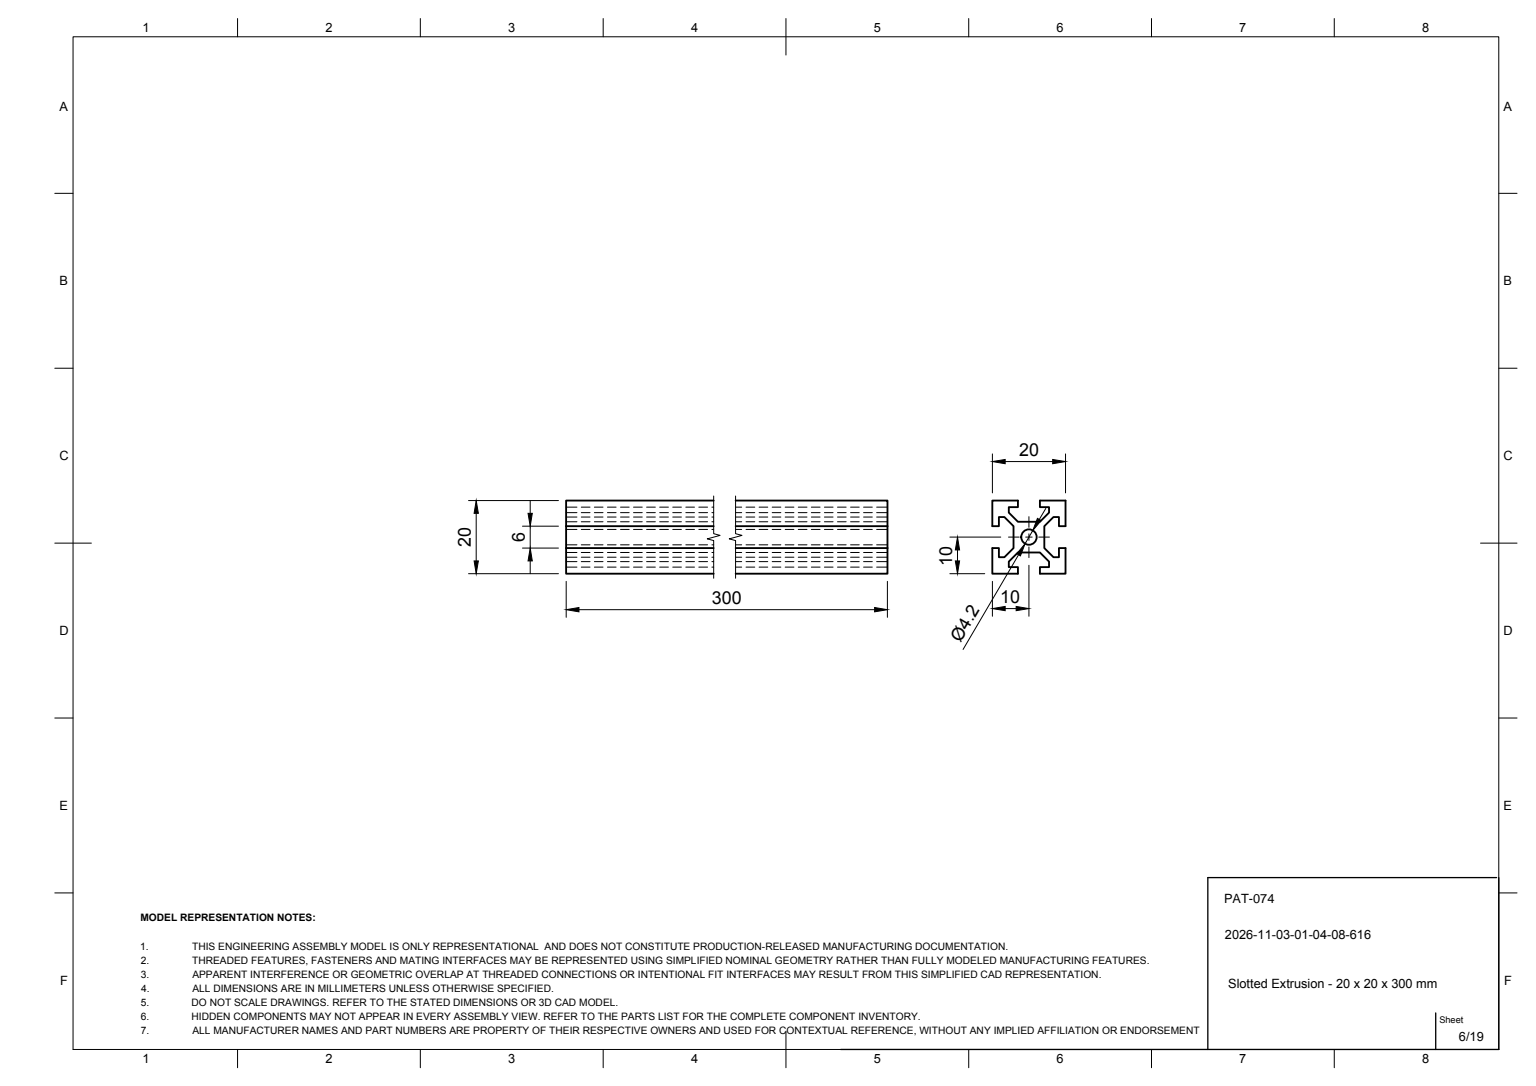
ISO-10303-21;
HEADER;
/* Generated by software containing ST-Developer
 * from STEP Tools, Inc. (www.steptools.com) 
 */

FILE_DESCRIPTION(
/* description */ ('Manual rail carriage with stops'),
/* implementation_level */ '2;1');

FILE_NAME(
/* name */ 'Slotted Extrusion - 20 x 20 x 300 mm.step',
/* time_stamp */ '2026-10-27T18:54:27-07:00',
/* author */ (''),
/* organization */ (''),
/* preprocessor_version */ 'ST-DEVELOPER v20.2',
/* originating_system */ 'Autodesk Translation Framework v15.17.0.0',
/* authorisation */ '');

FILE_SCHEMA (('AUTOMOTIVE_DESIGN { 1 0 10303 214 3 1 1 }'));
ENDSEC;

DATA;
#10=MECHANICAL_DESIGN_GEOMETRIC_PRESENTATION_REPRESENTATION('',(#274),#8499);
#238=SHAPE_REPRESENTATION_RELATIONSHIP('SRR','None',#8601,#256);
#256=ADVANCED_BREP_SHAPE_REPRESENTATION('',(#292),#8480);
#274=STYLED_ITEM('',(#8802),#292);
#292=MANIFOLD_SOLID_BREP('Body1',#4942);
#333=FACE_BOUND('',#936,.T.);
#334=FACE_BOUND('',#938,.T.);
#386=PLANE('',#5214);
#387=PLANE('',#5215);
#388=PLANE('',#5216);
#389=PLANE('',#5217);
#390=PLANE('',#5218);
#391=PLANE('',#5219);
#392=PLANE('',#5220);
#393=PLANE('',#5221);
#394=PLANE('',#5222);
#395=PLANE('',#5223);
#396=PLANE('',#5224);
#397=PLANE('',#5225);
#398=PLANE('',#5226);
#399=PLANE('',#5227);
#400=PLANE('',#5228);
#401=PLANE('',#5229);
#402=PLANE('',#5230);
#403=PLANE('',#5231);
#404=PLANE('',#5232);
#405=PLANE('',#5233);
#406=PLANE('',#5234);
#407=PLANE('',#5235);
#408=PLANE('',#5236);
#409=PLANE('',#5237);
#410=PLANE('',#5238);
#411=PLANE('',#5239);
#412=PLANE('',#5240);
#413=PLANE('',#5241);
#414=PLANE('',#5242);
#415=PLANE('',#5243);
#416=PLANE('',#5244);
#417=PLANE('',#5245);
#418=PLANE('',#5246);
#419=PLANE('',#5247);
#420=PLANE('',#5248);
#421=PLANE('',#5249);
#422=PLANE('',#5253);
#423=PLANE('',#5254);
#424=PLANE('',#5255);
#425=PLANE('',#5256);
#426=PLANE('',#5257);
#427=PLANE('',#5258);
#428=PLANE('',#5259);
#429=PLANE('',#5260);
#430=PLANE('',#5261);
#431=PLANE('',#5262);
#597=FACE_OUTER_BOUND('',#890,.T.);
#598=FACE_OUTER_BOUND('',#891,.T.);
#599=FACE_OUTER_BOUND('',#892,.T.);
#600=FACE_OUTER_BOUND('',#893,.T.);
#601=FACE_OUTER_BOUND('',#894,.T.);
#602=FACE_OUTER_BOUND('',#895,.T.);
#603=FACE_OUTER_BOUND('',#896,.T.);
#604=FACE_OUTER_BOUND('',#897,.T.);
#605=FACE_OUTER_BOUND('',#898,.T.);
#606=FACE_OUTER_BOUND('',#899,.T.);
#607=FACE_OUTER_BOUND('',#900,.T.);
#608=FACE_OUTER_BOUND('',#901,.T.);
#609=FACE_OUTER_BOUND('',#902,.T.);
#610=FACE_OUTER_BOUND('',#903,.T.);
#611=FACE_OUTER_BOUND('',#904,.T.);
#612=FACE_OUTER_BOUND('',#905,.T.);
#613=FACE_OUTER_BOUND('',#906,.T.);
#614=FACE_OUTER_BOUND('',#907,.T.);
#615=FACE_OUTER_BOUND('',#908,.T.);
#616=FACE_OUTER_BOUND('',#909,.T.);
#617=FACE_OUTER_BOUND('',#910,.T.);
#618=FACE_OUTER_BOUND('',#911,.T.);
#619=FACE_OUTER_BOUND('',#912,.T.);
#620=FACE_OUTER_BOUND('',#913,.T.);
#621=FACE_OUTER_BOUND('',#914,.T.);
#622=FACE_OUTER_BOUND('',#915,.T.);
#623=FACE_OUTER_BOUND('',#916,.T.);
#624=FACE_OUTER_BOUND('',#917,.T.);
#625=FACE_OUTER_BOUND('',#918,.T.);
#626=FACE_OUTER_BOUND('',#919,.T.);
#627=FACE_OUTER_BOUND('',#920,.T.);
#628=FACE_OUTER_BOUND('',#921,.T.);
#629=FACE_OUTER_BOUND('',#922,.T.);
#630=FACE_OUTER_BOUND('',#923,.T.);
#631=FACE_OUTER_BOUND('',#924,.T.);
#632=FACE_OUTER_BOUND('',#925,.T.);
#633=FACE_OUTER_BOUND('',#926,.T.);
#634=FACE_OUTER_BOUND('',#927,.T.);
#635=FACE_OUTER_BOUND('',#928,.T.);
#636=FACE_OUTER_BOUND('',#929,.T.);
#637=FACE_OUTER_BOUND('',#930,.T.);
#638=FACE_OUTER_BOUND('',#931,.T.);
#639=FACE_OUTER_BOUND('',#932,.T.);
#640=FACE_OUTER_BOUND('',#933,.T.);
#641=FACE_OUTER_BOUND('',#934,.T.);
#642=FACE_OUTER_BOUND('',#935,.T.);
#643=FACE_OUTER_BOUND('',#937,.T.);
#890=EDGE_LOOP('',(#3468,#3469,#3470,#3471));
#891=EDGE_LOOP('',(#3472,#3473,#3474,#3475));
#892=EDGE_LOOP('',(#3476,#3477,#3478,#3479));
#893=EDGE_LOOP('',(#3480,#3481,#3482,#3483));
#894=EDGE_LOOP('',(#3484,#3485,#3486,#3487));
#895=EDGE_LOOP('',(#3488,#3489,#3490,#3491));
#896=EDGE_LOOP('',(#3492,#3493,#3494,#3495));
#897=EDGE_LOOP('',(#3496,#3497,#3498,#3499));
#898=EDGE_LOOP('',(#3500,#3501,#3502,#3503));
#899=EDGE_LOOP('',(#3504,#3505,#3506,#3507));
#900=EDGE_LOOP('',(#3508,#3509,#3510,#3511));
#901=EDGE_LOOP('',(#3512,#3513,#3514,#3515));
#902=EDGE_LOOP('',(#3516,#3517,#3518,#3519));
#903=EDGE_LOOP('',(#3520,#3521,#3522,#3523));
#904=EDGE_LOOP('',(#3524,#3525,#3526,#3527));
#905=EDGE_LOOP('',(#3528,#3529,#3530,#3531));
#906=EDGE_LOOP('',(#3532,#3533,#3534,#3535));
#907=EDGE_LOOP('',(#3536,#3537,#3538,#3539));
#908=EDGE_LOOP('',(#3540,#3541,#3542,#3543));
#909=EDGE_LOOP('',(#3544,#3545,#3546,#3547));
#910=EDGE_LOOP('',(#3548,#3549,#3550,#3551));
#911=EDGE_LOOP('',(#3552,#3553,#3554,#3555));
#912=EDGE_LOOP('',(#3556,#3557,#3558,#3559));
#913=EDGE_LOOP('',(#3560,#3561,#3562,#3563));
#914=EDGE_LOOP('',(#3564,#3565,#3566,#3567));
#915=EDGE_LOOP('',(#3568,#3569,#3570,#3571));
#916=EDGE_LOOP('',(#3572,#3573,#3574,#3575));
#917=EDGE_LOOP('',(#3576,#3577,#3578,#3579));
#918=EDGE_LOOP('',(#3580,#3581,#3582,#3583));
#919=EDGE_LOOP('',(#3584,#3585,#3586,#3587));
#920=EDGE_LOOP('',(#3588,#3589,#3590,#3591));
#921=EDGE_LOOP('',(#3592,#3593,#3594,#3595));
#922=EDGE_LOOP('',(#3596,#3597,#3598,#3599));
#923=EDGE_LOOP('',(#3600,#3601,#3602,#3603));
#924=EDGE_LOOP('',(#3604,#3605,#3606,#3607));
#925=EDGE_LOOP('',(#3608,#3609,#3610,#3611));
#926=EDGE_LOOP('',(#3612,#3613,#3614,#3615));
#927=EDGE_LOOP('',(#3616,#3617,#3618,#3619));
#928=EDGE_LOOP('',(#3620,#3621,#3622,#3623));
#929=EDGE_LOOP('',(#3624,#3625,#3626,#3627));
#930=EDGE_LOOP('',(#3628,#3629,#3630,#3631));
#931=EDGE_LOOP('',(#3632,#3633,#3634,#3635));
#932=EDGE_LOOP('',(#3636,#3637,#3638,#3639));
#933=EDGE_LOOP('',(#3640,#3641,#3642,#3643));
#934=EDGE_LOOP('',(#3644,#3645,#3646,#3647));
#935=EDGE_LOOP('',(#3648,#3649,#3650,#3651,#3652,#3653,#3654,#3655,#3656,
#3657,#3658,#3659,#3660,#3661,#3662,#3663,#3664,#3665,#3666,#3667,#3668,
#3669,#3670,#3671,#3672,#3673,#3674,#3675,#3676,#3677,#3678,#3679,#3680,
#3681,#3682,#3683,#3684,#3685,#3686,#3687,#3688,#3689,#3690,#3691));
#936=EDGE_LOOP('',(#3692));
#937=EDGE_LOOP('',(#3693,#3694,#3695,#3696,#3697,#3698,#3699,#3700,#3701,
#3702,#3703,#3704,#3705,#3706,#3707,#3708,#3709,#3710,#3711,#3712,#3713,
#3714,#3715,#3716,#3717,#3718,#3719,#3720,#3721,#3722,#3723,#3724,#3725,
#3726,#3727,#3728,#3729,#3730,#3731,#3732,#3733,#3734,#3735,#3736));
#938=EDGE_LOOP('',(#3737));
#1208=LINE('',#7186,#1708);
#1209=LINE('',#7188,#1709);
#1210=LINE('',#7190,#1710);
#1211=LINE('',#7191,#1711);
#1212=LINE('',#7194,#1712);
#1213=LINE('',#7196,#1713);
#1214=LINE('',#7197,#1714);
#1215=LINE('',#7200,#1715);
#1216=LINE('',#7202,#1716);
#1217=LINE('',#7203,#1717);
#1218=LINE('',#7206,#1718);
#1219=LINE('',#7208,#1719);
#1220=LINE('',#7209,#1720);
#1221=LINE('',#7212,#1721);
#1222=LINE('',#7214,#1722);
#1223=LINE('',#7215,#1723);
#1224=LINE('',#7218,#1724);
#1225=LINE('',#7220,#1725);
#1226=LINE('',#7221,#1726);
#1227=LINE('',#7224,#1727);
#1228=LINE('',#7226,#1728);
#1229=LINE('',#7227,#1729);
#1230=LINE('',#7230,#1730);
#1231=LINE('',#7232,#1731);
#1232=LINE('',#7233,#1732);
#1233=LINE('',#7236,#1733);
#1234=LINE('',#7238,#1734);
#1235=LINE('',#7239,#1735);
#1236=LINE('',#7243,#1736);
#1237=LINE('',#7245,#1737);
#1238=LINE('',#7247,#1738);
#1239=LINE('',#7248,#1739);
#1240=LINE('',#7251,#1740);
#1241=LINE('',#7253,#1741);
#1242=LINE('',#7254,#1742);
#1243=LINE('',#7257,#1743);
#1244=LINE('',#7259,#1744);
#1245=LINE('',#7260,#1745);
#1246=LINE('',#7263,#1746);
#1247=LINE('',#7265,#1747);
#1248=LINE('',#7266,#1748);
#1249=LINE('',#7269,#1749);
#1250=LINE('',#7271,#1750);
#1251=LINE('',#7272,#1751);
#1252=LINE('',#7275,#1752);
#1253=LINE('',#7277,#1753);
#1254=LINE('',#7278,#1754);
#1255=LINE('',#7281,#1755);
#1256=LINE('',#7283,#1756);
#1257=LINE('',#7284,#1757);
#1258=LINE('',#7287,#1758);
#1259=LINE('',#7289,#1759);
#1260=LINE('',#7290,#1760);
#1261=LINE('',#7293,#1761);
#1262=LINE('',#7295,#1762);
#1263=LINE('',#7296,#1763);
#1264=LINE('',#7300,#1764);
#1265=LINE('',#7302,#1765);
#1266=LINE('',#7304,#1766);
#1267=LINE('',#7305,#1767);
#1268=LINE('',#7308,#1768);
#1269=LINE('',#7310,#1769);
#1270=LINE('',#7311,#1770);
#1271=LINE('',#7314,#1771);
#1272=LINE('',#7316,#1772);
#1273=LINE('',#7317,#1773);
#1274=LINE('',#7320,#1774);
#1275=LINE('',#7322,#1775);
#1276=LINE('',#7323,#1776);
#1277=LINE('',#7326,#1777);
#1278=LINE('',#7328,#1778);
#1279=LINE('',#7329,#1779);
#1280=LINE('',#7332,#1780);
#1281=LINE('',#7334,#1781);
#1282=LINE('',#7335,#1782);
#1283=LINE('',#7338,#1783);
#1284=LINE('',#7340,#1784);
#1285=LINE('',#7341,#1785);
#1286=LINE('',#7344,#1786);
#1287=LINE('',#7346,#1787);
#1288=LINE('',#7347,#1788);
#1289=LINE('',#7350,#1789);
#1290=LINE('',#7352,#1790);
#1291=LINE('',#7353,#1791);
#1292=LINE('',#7357,#1792);
#1293=LINE('',#7359,#1793);
#1294=LINE('',#7361,#1794);
#1295=LINE('',#7362,#1795);
#1296=LINE('',#7365,#1796);
#1297=LINE('',#7367,#1797);
#1298=LINE('',#7368,#1798);
#1299=LINE('',#7371,#1799);
#1300=LINE('',#7373,#1800);
#1301=LINE('',#7374,#1801);
#1302=LINE('',#7377,#1802);
#1303=LINE('',#7379,#1803);
#1304=LINE('',#7380,#1804);
#1305=LINE('',#7383,#1805);
#1306=LINE('',#7385,#1806);
#1307=LINE('',#7386,#1807);
#1308=LINE('',#7389,#1808);
#1309=LINE('',#7391,#1809);
#1310=LINE('',#7392,#1810);
#1311=LINE('',#7395,#1811);
#1312=LINE('',#7397,#1812);
#1313=LINE('',#7398,#1813);
#1314=LINE('',#7401,#1814);
#1315=LINE('',#7403,#1815);
#1316=LINE('',#7404,#1816);
#1317=LINE('',#7407,#1817);
#1318=LINE('',#7409,#1818);
#1319=LINE('',#7410,#1819);
#1320=LINE('',#7415,#1820);
#1321=LINE('',#7419,#1821);
#1322=LINE('',#7421,#1822);
#1323=LINE('',#7422,#1823);
#1324=LINE('',#7425,#1824);
#1325=LINE('',#7427,#1825);
#1326=LINE('',#7428,#1826);
#1327=LINE('',#7430,#1827);
#1328=LINE('',#7431,#1828);
#1329=LINE('',#7434,#1829);
#1330=LINE('',#7436,#1830);
#1331=LINE('',#7437,#1831);
#1332=LINE('',#7439,#1832);
#1333=LINE('',#7440,#1833);
#1334=LINE('',#7443,#1834);
#1335=LINE('',#7445,#1835);
#1336=LINE('',#7446,#1836);
#1337=LINE('',#7448,#1837);
#1338=LINE('',#7449,#1838);
#1339=LINE('',#7451,#1839);
#1340=LINE('',#7452,#1840);
#1708=VECTOR('',#5763,1.);
#1709=VECTOR('',#5764,1.);
#1710=VECTOR('',#5765,1.);
#1711=VECTOR('',#5766,1.);
#1712=VECTOR('',#5769,1.);
#1713=VECTOR('',#5770,1.);
#1714=VECTOR('',#5771,1.);
#1715=VECTOR('',#5774,1.);
#1716=VECTOR('',#5775,1.);
#1717=VECTOR('',#5776,1.);
#1718=VECTOR('',#5779,1.);
#1719=VECTOR('',#5780,1.);
#1720=VECTOR('',#5781,1.);
#1721=VECTOR('',#5784,1.);
#1722=VECTOR('',#5785,1.);
#1723=VECTOR('',#5786,1.);
#1724=VECTOR('',#5789,1.);
#1725=VECTOR('',#5790,1.);
#1726=VECTOR('',#5791,1.);
#1727=VECTOR('',#5794,1.);
#1728=VECTOR('',#5795,1.);
#1729=VECTOR('',#5796,1.);
#1730=VECTOR('',#5799,1.);
#1731=VECTOR('',#5800,1.);
#1732=VECTOR('',#5801,1.);
#1733=VECTOR('',#5804,1.);
#1734=VECTOR('',#5805,1.);
#1735=VECTOR('',#5806,1.);
#1736=VECTOR('',#5809,1.);
#1737=VECTOR('',#5810,1.);
#1738=VECTOR('',#5811,1.);
#1739=VECTOR('',#5812,1.);
#1740=VECTOR('',#5815,1.);
#1741=VECTOR('',#5816,1.);
#1742=VECTOR('',#5817,1.);
#1743=VECTOR('',#5820,1.);
#1744=VECTOR('',#5821,1.);
#1745=VECTOR('',#5822,1.);
#1746=VECTOR('',#5825,1.);
#1747=VECTOR('',#5826,1.);
#1748=VECTOR('',#5827,1.);
#1749=VECTOR('',#5830,1.);
#1750=VECTOR('',#5831,1.);
#1751=VECTOR('',#5832,1.);
#1752=VECTOR('',#5835,1.);
#1753=VECTOR('',#5836,1.);
#1754=VECTOR('',#5837,1.);
#1755=VECTOR('',#5840,1.);
#1756=VECTOR('',#5841,1.);
#1757=VECTOR('',#5842,1.);
#1758=VECTOR('',#5845,1.);
#1759=VECTOR('',#5846,1.);
#1760=VECTOR('',#5847,1.);
#1761=VECTOR('',#5850,1.);
#1762=VECTOR('',#5851,1.);
#1763=VECTOR('',#5852,1.);
#1764=VECTOR('',#5855,1.);
#1765=VECTOR('',#5856,1.);
#1766=VECTOR('',#5857,1.);
#1767=VECTOR('',#5858,1.);
#1768=VECTOR('',#5861,1.);
#1769=VECTOR('',#5862,1.);
#1770=VECTOR('',#5863,1.);
#1771=VECTOR('',#5866,1.);
#1772=VECTOR('',#5867,1.);
#1773=VECTOR('',#5868,1.);
#1774=VECTOR('',#5871,1.);
#1775=VECTOR('',#5872,1.);
#1776=VECTOR('',#5873,1.);
#1777=VECTOR('',#5876,1.);
#1778=VECTOR('',#5877,1.);
#1779=VECTOR('',#5878,1.);
#1780=VECTOR('',#5881,1.);
#1781=VECTOR('',#5882,1.);
#1782=VECTOR('',#5883,1.);
#1783=VECTOR('',#5886,1.);
#1784=VECTOR('',#5887,1.);
#1785=VECTOR('',#5888,1.);
#1786=VECTOR('',#5891,1.);
#1787=VECTOR('',#5892,1.);
#1788=VECTOR('',#5893,1.);
#1789=VECTOR('',#5896,1.);
#1790=VECTOR('',#5897,1.);
#1791=VECTOR('',#5898,1.);
#1792=VECTOR('',#5901,1.);
#1793=VECTOR('',#5902,1.);
#1794=VECTOR('',#5903,1.);
#1795=VECTOR('',#5904,1.);
#1796=VECTOR('',#5907,1.);
#1797=VECTOR('',#5908,1.);
#1798=VECTOR('',#5909,1.);
#1799=VECTOR('',#5912,1.);
#1800=VECTOR('',#5913,1.);
#1801=VECTOR('',#5914,1.);
#1802=VECTOR('',#5917,1.);
#1803=VECTOR('',#5918,1.);
#1804=VECTOR('',#5919,1.);
#1805=VECTOR('',#5922,1.);
#1806=VECTOR('',#5923,1.);
#1807=VECTOR('',#5924,1.);
#1808=VECTOR('',#5927,1.);
#1809=VECTOR('',#5928,1.);
#1810=VECTOR('',#5929,1.);
#1811=VECTOR('',#5932,1.);
#1812=VECTOR('',#5933,1.);
#1813=VECTOR('',#5934,1.);
#1814=VECTOR('',#5937,1.);
#1815=VECTOR('',#5938,1.);
#1816=VECTOR('',#5939,1.);
#1817=VECTOR('',#5942,1.);
#1818=VECTOR('',#5943,1.);
#1819=VECTOR('',#5944,1.);
#1820=VECTOR('',#5949,0.21);
#1821=VECTOR('',#5954,1.);
#1822=VECTOR('',#5955,1.);
#1823=VECTOR('',#5956,1.);
#1824=VECTOR('',#5959,1.);
#1825=VECTOR('',#5960,1.);
#1826=VECTOR('',#5961,1.);
#1827=VECTOR('',#5964,1.);
#1828=VECTOR('',#5965,1.);
#1829=VECTOR('',#5968,1.);
#1830=VECTOR('',#5969,1.);
#1831=VECTOR('',#5970,1.);
#1832=VECTOR('',#5973,1.);
#1833=VECTOR('',#5974,1.);
#1834=VECTOR('',#5977,1.);
#1835=VECTOR('',#5978,1.);
#1836=VECTOR('',#5979,1.);
#1837=VECTOR('',#5982,1.);
#1838=VECTOR('',#5983,1.);
#1839=VECTOR('',#5986,1.);
#1840=VECTOR('',#5987,1.);
#2210=CIRCLE('',#5251,0.21);
#2211=CIRCLE('',#5252,0.21);
#2348=VERTEX_POINT('',#7184);
#2349=VERTEX_POINT('',#7185);
#2350=VERTEX_POINT('',#7187);
#2351=VERTEX_POINT('',#7189);
#2352=VERTEX_POINT('',#7193);
#2353=VERTEX_POINT('',#7195);
#2354=VERTEX_POINT('',#7199);
#2355=VERTEX_POINT('',#7201);
#2356=VERTEX_POINT('',#7205);
#2357=VERTEX_POINT('',#7207);
#2358=VERTEX_POINT('',#7211);
#2359=VERTEX_POINT('',#7213);
#2360=VERTEX_POINT('',#7217);
#2361=VERTEX_POINT('',#7219);
#2362=VERTEX_POINT('',#7223);
#2363=VERTEX_POINT('',#7225);
#2364=VERTEX_POINT('',#7229);
#2365=VERTEX_POINT('',#7231);
#2366=VERTEX_POINT('',#7235);
#2367=VERTEX_POINT('',#7237);
#2368=VERTEX_POINT('',#7241);
#2369=VERTEX_POINT('',#7242);
#2370=VERTEX_POINT('',#7244);
#2371=VERTEX_POINT('',#7246);
#2372=VERTEX_POINT('',#7250);
#2373=VERTEX_POINT('',#7252);
#2374=VERTEX_POINT('',#7256);
#2375=VERTEX_POINT('',#7258);
#2376=VERTEX_POINT('',#7262);
#2377=VERTEX_POINT('',#7264);
#2378=VERTEX_POINT('',#7268);
#2379=VERTEX_POINT('',#7270);
#2380=VERTEX_POINT('',#7274);
#2381=VERTEX_POINT('',#7276);
#2382=VERTEX_POINT('',#7280);
#2383=VERTEX_POINT('',#7282);
#2384=VERTEX_POINT('',#7286);
#2385=VERTEX_POINT('',#7288);
#2386=VERTEX_POINT('',#7292);
#2387=VERTEX_POINT('',#7294);
#2388=VERTEX_POINT('',#7298);
#2389=VERTEX_POINT('',#7299);
#2390=VERTEX_POINT('',#7301);
#2391=VERTEX_POINT('',#7303);
#2392=VERTEX_POINT('',#7307);
#2393=VERTEX_POINT('',#7309);
#2394=VERTEX_POINT('',#7313);
#2395=VERTEX_POINT('',#7315);
#2396=VERTEX_POINT('',#7319);
#2397=VERTEX_POINT('',#7321);
#2398=VERTEX_POINT('',#7325);
#2399=VERTEX_POINT('',#7327);
#2400=VERTEX_POINT('',#7331);
#2401=VERTEX_POINT('',#7333);
#2402=VERTEX_POINT('',#7337);
#2403=VERTEX_POINT('',#7339);
#2404=VERTEX_POINT('',#7343);
#2405=VERTEX_POINT('',#7345);
#2406=VERTEX_POINT('',#7349);
#2407=VERTEX_POINT('',#7351);
#2408=VERTEX_POINT('',#7355);
#2409=VERTEX_POINT('',#7356);
#2410=VERTEX_POINT('',#7358);
#2411=VERTEX_POINT('',#7360);
#2412=VERTEX_POINT('',#7364);
#2413=VERTEX_POINT('',#7366);
#2414=VERTEX_POINT('',#7370);
#2415=VERTEX_POINT('',#7372);
#2416=VERTEX_POINT('',#7376);
#2417=VERTEX_POINT('',#7378);
#2418=VERTEX_POINT('',#7382);
#2419=VERTEX_POINT('',#7384);
#2420=VERTEX_POINT('',#7388);
#2421=VERTEX_POINT('',#7390);
#2422=VERTEX_POINT('',#7394);
#2423=VERTEX_POINT('',#7396);
#2424=VERTEX_POINT('',#7400);
#2425=VERTEX_POINT('',#7402);
#2426=VERTEX_POINT('',#7406);
#2427=VERTEX_POINT('',#7408);
#2428=VERTEX_POINT('',#7412);
#2429=VERTEX_POINT('',#7414);
#2430=VERTEX_POINT('',#7418);
#2431=VERTEX_POINT('',#7420);
#2432=VERTEX_POINT('',#7424);
#2433=VERTEX_POINT('',#7426);
#2434=VERTEX_POINT('',#7433);
#2435=VERTEX_POINT('',#7435);
#2436=VERTEX_POINT('',#7442);
#2437=VERTEX_POINT('',#7444);
#2782=EDGE_CURVE('',#2348,#2349,#1208,.T.);
#2783=EDGE_CURVE('',#2348,#2350,#1209,.T.);
#2784=EDGE_CURVE('',#2351,#2350,#1210,.T.);
#2785=EDGE_CURVE('',#2349,#2351,#1211,.T.);
#2786=EDGE_CURVE('',#2352,#2348,#1212,.T.);
#2787=EDGE_CURVE('',#2352,#2353,#1213,.T.);
#2788=EDGE_CURVE('',#2350,#2353,#1214,.T.);
#2789=EDGE_CURVE('',#2354,#2352,#1215,.T.);
#2790=EDGE_CURVE('',#2354,#2355,#1216,.T.);
#2791=EDGE_CURVE('',#2353,#2355,#1217,.T.);
#2792=EDGE_CURVE('',#2356,#2354,#1218,.T.);
#2793=EDGE_CURVE('',#2356,#2357,#1219,.T.);
#2794=EDGE_CURVE('',#2355,#2357,#1220,.T.);
#2795=EDGE_CURVE('',#2358,#2356,#1221,.T.);
#2796=EDGE_CURVE('',#2358,#2359,#1222,.T.);
#2797=EDGE_CURVE('',#2357,#2359,#1223,.T.);
#2798=EDGE_CURVE('',#2360,#2358,#1224,.T.);
#2799=EDGE_CURVE('',#2360,#2361,#1225,.T.);
#2800=EDGE_CURVE('',#2359,#2361,#1226,.T.);
#2801=EDGE_CURVE('',#2362,#2360,#1227,.T.);
#2802=EDGE_CURVE('',#2362,#2363,#1228,.T.);
#2803=EDGE_CURVE('',#2361,#2363,#1229,.T.);
#2804=EDGE_CURVE('',#2364,#2362,#1230,.T.);
#2805=EDGE_CURVE('',#2364,#2365,#1231,.T.);
#2806=EDGE_CURVE('',#2363,#2365,#1232,.T.);
#2807=EDGE_CURVE('',#2366,#2364,#1233,.T.);
#2808=EDGE_CURVE('',#2367,#2366,#1234,.T.);
#2809=EDGE_CURVE('',#2365,#2367,#1235,.T.);
#2810=EDGE_CURVE('',#2368,#2369,#1236,.T.);
#2811=EDGE_CURVE('',#2368,#2370,#1237,.T.);
#2812=EDGE_CURVE('',#2371,#2370,#1238,.T.);
#2813=EDGE_CURVE('',#2369,#2371,#1239,.T.);
#2814=EDGE_CURVE('',#2372,#2368,#1240,.T.);
#2815=EDGE_CURVE('',#2372,#2373,#1241,.T.);
#2816=EDGE_CURVE('',#2370,#2373,#1242,.T.);
#2817=EDGE_CURVE('',#2374,#2372,#1243,.T.);
#2818=EDGE_CURVE('',#2374,#2375,#1244,.T.);
#2819=EDGE_CURVE('',#2373,#2375,#1245,.T.);
#2820=EDGE_CURVE('',#2376,#2374,#1246,.T.);
#2821=EDGE_CURVE('',#2376,#2377,#1247,.T.);
#2822=EDGE_CURVE('',#2375,#2377,#1248,.T.);
#2823=EDGE_CURVE('',#2378,#2376,#1249,.T.);
#2824=EDGE_CURVE('',#2378,#2379,#1250,.T.);
#2825=EDGE_CURVE('',#2377,#2379,#1251,.T.);
#2826=EDGE_CURVE('',#2380,#2378,#1252,.T.);
#2827=EDGE_CURVE('',#2380,#2381,#1253,.T.);
#2828=EDGE_CURVE('',#2379,#2381,#1254,.T.);
#2829=EDGE_CURVE('',#2382,#2380,#1255,.T.);
#2830=EDGE_CURVE('',#2382,#2383,#1256,.T.);
#2831=EDGE_CURVE('',#2381,#2383,#1257,.T.);
#2832=EDGE_CURVE('',#2384,#2382,#1258,.T.);
#2833=EDGE_CURVE('',#2384,#2385,#1259,.T.);
#2834=EDGE_CURVE('',#2383,#2385,#1260,.T.);
#2835=EDGE_CURVE('',#2386,#2384,#1261,.T.);
#2836=EDGE_CURVE('',#2387,#2386,#1262,.T.);
#2837=EDGE_CURVE('',#2385,#2387,#1263,.T.);
#2838=EDGE_CURVE('',#2388,#2389,#1264,.T.);
#2839=EDGE_CURVE('',#2388,#2390,#1265,.T.);
#2840=EDGE_CURVE('',#2391,#2390,#1266,.T.);
#2841=EDGE_CURVE('',#2389,#2391,#1267,.T.);
#2842=EDGE_CURVE('',#2392,#2388,#1268,.T.);
#2843=EDGE_CURVE('',#2392,#2393,#1269,.T.);
#2844=EDGE_CURVE('',#2390,#2393,#1270,.T.);
#2845=EDGE_CURVE('',#2394,#2392,#1271,.T.);
#2846=EDGE_CURVE('',#2394,#2395,#1272,.T.);
#2847=EDGE_CURVE('',#2393,#2395,#1273,.T.);
#2848=EDGE_CURVE('',#2396,#2394,#1274,.T.);
#2849=EDGE_CURVE('',#2396,#2397,#1275,.T.);
#2850=EDGE_CURVE('',#2395,#2397,#1276,.T.);
#2851=EDGE_CURVE('',#2398,#2396,#1277,.T.);
#2852=EDGE_CURVE('',#2398,#2399,#1278,.T.);
#2853=EDGE_CURVE('',#2397,#2399,#1279,.T.);
#2854=EDGE_CURVE('',#2400,#2398,#1280,.T.);
#2855=EDGE_CURVE('',#2400,#2401,#1281,.T.);
#2856=EDGE_CURVE('',#2399,#2401,#1282,.T.);
#2857=EDGE_CURVE('',#2402,#2400,#1283,.T.);
#2858=EDGE_CURVE('',#2402,#2403,#1284,.T.);
#2859=EDGE_CURVE('',#2401,#2403,#1285,.T.);
#2860=EDGE_CURVE('',#2404,#2402,#1286,.T.);
#2861=EDGE_CURVE('',#2404,#2405,#1287,.T.);
#2862=EDGE_CURVE('',#2403,#2405,#1288,.T.);
#2863=EDGE_CURVE('',#2406,#2404,#1289,.T.);
#2864=EDGE_CURVE('',#2407,#2406,#1290,.T.);
#2865=EDGE_CURVE('',#2405,#2407,#1291,.T.);
#2866=EDGE_CURVE('',#2408,#2409,#1292,.T.);
#2867=EDGE_CURVE('',#2408,#2410,#1293,.T.);
#2868=EDGE_CURVE('',#2411,#2410,#1294,.T.);
#2869=EDGE_CURVE('',#2409,#2411,#1295,.T.);
#2870=EDGE_CURVE('',#2412,#2408,#1296,.T.);
#2871=EDGE_CURVE('',#2412,#2413,#1297,.T.);
#2872=EDGE_CURVE('',#2410,#2413,#1298,.T.);
#2873=EDGE_CURVE('',#2414,#2412,#1299,.T.);
#2874=EDGE_CURVE('',#2414,#2415,#1300,.T.);
#2875=EDGE_CURVE('',#2413,#2415,#1301,.T.);
#2876=EDGE_CURVE('',#2416,#2414,#1302,.T.);
#2877=EDGE_CURVE('',#2416,#2417,#1303,.T.);
#2878=EDGE_CURVE('',#2415,#2417,#1304,.T.);
#2879=EDGE_CURVE('',#2418,#2416,#1305,.T.);
#2880=EDGE_CURVE('',#2418,#2419,#1306,.T.);
#2881=EDGE_CURVE('',#2417,#2419,#1307,.T.);
#2882=EDGE_CURVE('',#2420,#2418,#1308,.T.);
#2883=EDGE_CURVE('',#2420,#2421,#1309,.T.);
#2884=EDGE_CURVE('',#2419,#2421,#1310,.T.);
#2885=EDGE_CURVE('',#2422,#2420,#1311,.T.);
#2886=EDGE_CURVE('',#2422,#2423,#1312,.T.);
#2887=EDGE_CURVE('',#2421,#2423,#1313,.T.);
#2888=EDGE_CURVE('',#2424,#2422,#1314,.T.);
#2889=EDGE_CURVE('',#2424,#2425,#1315,.T.);
#2890=EDGE_CURVE('',#2423,#2425,#1316,.T.);
#2891=EDGE_CURVE('',#2426,#2424,#1317,.T.);
#2892=EDGE_CURVE('',#2427,#2426,#1318,.T.);
#2893=EDGE_CURVE('',#2425,#2427,#1319,.T.);
#2894=EDGE_CURVE('',#2428,#2428,#2210,.T.);
#2895=EDGE_CURVE('',#2428,#2429,#1320,.T.);
#2896=EDGE_CURVE('',#2429,#2429,#2211,.T.);
#2897=EDGE_CURVE('',#2366,#2430,#1321,.T.);
#2898=EDGE_CURVE('',#2430,#2431,#1322,.T.);
#2899=EDGE_CURVE('',#2367,#2431,#1323,.T.);
#2900=EDGE_CURVE('',#2432,#2351,#1324,.T.);
#2901=EDGE_CURVE('',#2433,#2432,#1325,.T.);
#2902=EDGE_CURVE('',#2433,#2349,#1326,.T.);
#2903=EDGE_CURVE('',#2386,#2433,#1327,.T.);
#2904=EDGE_CURVE('',#2387,#2432,#1328,.T.);
#2905=EDGE_CURVE('',#2434,#2371,#1329,.T.);
#2906=EDGE_CURVE('',#2435,#2434,#1330,.T.);
#2907=EDGE_CURVE('',#2435,#2369,#1331,.T.);
#2908=EDGE_CURVE('',#2406,#2435,#1332,.T.);
#2909=EDGE_CURVE('',#2407,#2434,#1333,.T.);
#2910=EDGE_CURVE('',#2436,#2391,#1334,.T.);
#2911=EDGE_CURVE('',#2437,#2436,#1335,.T.);
#2912=EDGE_CURVE('',#2437,#2389,#1336,.T.);
#2913=EDGE_CURVE('',#2426,#2437,#1337,.T.);
#2914=EDGE_CURVE('',#2427,#2436,#1338,.T.);
#2915=EDGE_CURVE('',#2431,#2411,#1339,.T.);
#2916=EDGE_CURVE('',#2430,#2409,#1340,.T.);
#3468=ORIENTED_EDGE('',*,*,#2782,.F.);
#3469=ORIENTED_EDGE('',*,*,#2783,.T.);
#3470=ORIENTED_EDGE('',*,*,#2784,.F.);
#3471=ORIENTED_EDGE('',*,*,#2785,.F.);
#3472=ORIENTED_EDGE('',*,*,#2786,.F.);
#3473=ORIENTED_EDGE('',*,*,#2787,.T.);
#3474=ORIENTED_EDGE('',*,*,#2788,.F.);
#3475=ORIENTED_EDGE('',*,*,#2783,.F.);
#3476=ORIENTED_EDGE('',*,*,#2789,.F.);
#3477=ORIENTED_EDGE('',*,*,#2790,.T.);
#3478=ORIENTED_EDGE('',*,*,#2791,.F.);
#3479=ORIENTED_EDGE('',*,*,#2787,.F.);
#3480=ORIENTED_EDGE('',*,*,#2792,.F.);
#3481=ORIENTED_EDGE('',*,*,#2793,.T.);
#3482=ORIENTED_EDGE('',*,*,#2794,.F.);
#3483=ORIENTED_EDGE('',*,*,#2790,.F.);
#3484=ORIENTED_EDGE('',*,*,#2795,.F.);
#3485=ORIENTED_EDGE('',*,*,#2796,.T.);
#3486=ORIENTED_EDGE('',*,*,#2797,.F.);
#3487=ORIENTED_EDGE('',*,*,#2793,.F.);
#3488=ORIENTED_EDGE('',*,*,#2798,.F.);
#3489=ORIENTED_EDGE('',*,*,#2799,.T.);
#3490=ORIENTED_EDGE('',*,*,#2800,.F.);
#3491=ORIENTED_EDGE('',*,*,#2796,.F.);
#3492=ORIENTED_EDGE('',*,*,#2801,.F.);
#3493=ORIENTED_EDGE('',*,*,#2802,.T.);
#3494=ORIENTED_EDGE('',*,*,#2803,.F.);
#3495=ORIENTED_EDGE('',*,*,#2799,.F.);
#3496=ORIENTED_EDGE('',*,*,#2804,.F.);
#3497=ORIENTED_EDGE('',*,*,#2805,.T.);
#3498=ORIENTED_EDGE('',*,*,#2806,.F.);
#3499=ORIENTED_EDGE('',*,*,#2802,.F.);
#3500=ORIENTED_EDGE('',*,*,#2807,.F.);
#3501=ORIENTED_EDGE('',*,*,#2808,.F.);
#3502=ORIENTED_EDGE('',*,*,#2809,.F.);
#3503=ORIENTED_EDGE('',*,*,#2805,.F.);
#3504=ORIENTED_EDGE('',*,*,#2810,.F.);
#3505=ORIENTED_EDGE('',*,*,#2811,.T.);
#3506=ORIENTED_EDGE('',*,*,#2812,.F.);
#3507=ORIENTED_EDGE('',*,*,#2813,.F.);
#3508=ORIENTED_EDGE('',*,*,#2814,.F.);
#3509=ORIENTED_EDGE('',*,*,#2815,.T.);
#3510=ORIENTED_EDGE('',*,*,#2816,.F.);
#3511=ORIENTED_EDGE('',*,*,#2811,.F.);
#3512=ORIENTED_EDGE('',*,*,#2817,.F.);
#3513=ORIENTED_EDGE('',*,*,#2818,.T.);
#3514=ORIENTED_EDGE('',*,*,#2819,.F.);
#3515=ORIENTED_EDGE('',*,*,#2815,.F.);
#3516=ORIENTED_EDGE('',*,*,#2820,.F.);
#3517=ORIENTED_EDGE('',*,*,#2821,.T.);
#3518=ORIENTED_EDGE('',*,*,#2822,.F.);
#3519=ORIENTED_EDGE('',*,*,#2818,.F.);
#3520=ORIENTED_EDGE('',*,*,#2823,.F.);
#3521=ORIENTED_EDGE('',*,*,#2824,.T.);
#3522=ORIENTED_EDGE('',*,*,#2825,.F.);
#3523=ORIENTED_EDGE('',*,*,#2821,.F.);
#3524=ORIENTED_EDGE('',*,*,#2826,.F.);
#3525=ORIENTED_EDGE('',*,*,#2827,.T.);
#3526=ORIENTED_EDGE('',*,*,#2828,.F.);
#3527=ORIENTED_EDGE('',*,*,#2824,.F.);
#3528=ORIENTED_EDGE('',*,*,#2829,.F.);
#3529=ORIENTED_EDGE('',*,*,#2830,.T.);
#3530=ORIENTED_EDGE('',*,*,#2831,.F.);
#3531=ORIENTED_EDGE('',*,*,#2827,.F.);
#3532=ORIENTED_EDGE('',*,*,#2832,.F.);
#3533=ORIENTED_EDGE('',*,*,#2833,.T.);
#3534=ORIENTED_EDGE('',*,*,#2834,.F.);
#3535=ORIENTED_EDGE('',*,*,#2830,.F.);
#3536=ORIENTED_EDGE('',*,*,#2835,.F.);
#3537=ORIENTED_EDGE('',*,*,#2836,.F.);
#3538=ORIENTED_EDGE('',*,*,#2837,.F.);
#3539=ORIENTED_EDGE('',*,*,#2833,.F.);
#3540=ORIENTED_EDGE('',*,*,#2838,.F.);
#3541=ORIENTED_EDGE('',*,*,#2839,.T.);
#3542=ORIENTED_EDGE('',*,*,#2840,.F.);
#3543=ORIENTED_EDGE('',*,*,#2841,.F.);
#3544=ORIENTED_EDGE('',*,*,#2842,.F.);
#3545=ORIENTED_EDGE('',*,*,#2843,.T.);
#3546=ORIENTED_EDGE('',*,*,#2844,.F.);
#3547=ORIENTED_EDGE('',*,*,#2839,.F.);
#3548=ORIENTED_EDGE('',*,*,#2845,.F.);
#3549=ORIENTED_EDGE('',*,*,#2846,.T.);
#3550=ORIENTED_EDGE('',*,*,#2847,.F.);
#3551=ORIENTED_EDGE('',*,*,#2843,.F.);
#3552=ORIENTED_EDGE('',*,*,#2848,.F.);
#3553=ORIENTED_EDGE('',*,*,#2849,.T.);
#3554=ORIENTED_EDGE('',*,*,#2850,.F.);
#3555=ORIENTED_EDGE('',*,*,#2846,.F.);
#3556=ORIENTED_EDGE('',*,*,#2851,.F.);
#3557=ORIENTED_EDGE('',*,*,#2852,.T.);
#3558=ORIENTED_EDGE('',*,*,#2853,.F.);
#3559=ORIENTED_EDGE('',*,*,#2849,.F.);
#3560=ORIENTED_EDGE('',*,*,#2854,.F.);
#3561=ORIENTED_EDGE('',*,*,#2855,.T.);
#3562=ORIENTED_EDGE('',*,*,#2856,.F.);
#3563=ORIENTED_EDGE('',*,*,#2852,.F.);
#3564=ORIENTED_EDGE('',*,*,#2857,.F.);
#3565=ORIENTED_EDGE('',*,*,#2858,.T.);
#3566=ORIENTED_EDGE('',*,*,#2859,.F.);
#3567=ORIENTED_EDGE('',*,*,#2855,.F.);
#3568=ORIENTED_EDGE('',*,*,#2860,.F.);
#3569=ORIENTED_EDGE('',*,*,#2861,.T.);
#3570=ORIENTED_EDGE('',*,*,#2862,.F.);
#3571=ORIENTED_EDGE('',*,*,#2858,.F.);
#3572=ORIENTED_EDGE('',*,*,#2863,.F.);
#3573=ORIENTED_EDGE('',*,*,#2864,.F.);
#3574=ORIENTED_EDGE('',*,*,#2865,.F.);
#3575=ORIENTED_EDGE('',*,*,#2861,.F.);
#3576=ORIENTED_EDGE('',*,*,#2866,.F.);
#3577=ORIENTED_EDGE('',*,*,#2867,.T.);
#3578=ORIENTED_EDGE('',*,*,#2868,.F.);
#3579=ORIENTED_EDGE('',*,*,#2869,.F.);
#3580=ORIENTED_EDGE('',*,*,#2870,.F.);
#3581=ORIENTED_EDGE('',*,*,#2871,.T.);
#3582=ORIENTED_EDGE('',*,*,#2872,.F.);
#3583=ORIENTED_EDGE('',*,*,#2867,.F.);
#3584=ORIENTED_EDGE('',*,*,#2873,.F.);
#3585=ORIENTED_EDGE('',*,*,#2874,.T.);
#3586=ORIENTED_EDGE('',*,*,#2875,.F.);
#3587=ORIENTED_EDGE('',*,*,#2871,.F.);
#3588=ORIENTED_EDGE('',*,*,#2876,.F.);
#3589=ORIENTED_EDGE('',*,*,#2877,.T.);
#3590=ORIENTED_EDGE('',*,*,#2878,.F.);
#3591=ORIENTED_EDGE('',*,*,#2874,.F.);
#3592=ORIENTED_EDGE('',*,*,#2879,.F.);
#3593=ORIENTED_EDGE('',*,*,#2880,.T.);
#3594=ORIENTED_EDGE('',*,*,#2881,.F.);
#3595=ORIENTED_EDGE('',*,*,#2877,.F.);
#3596=ORIENTED_EDGE('',*,*,#2882,.F.);
#3597=ORIENTED_EDGE('',*,*,#2883,.T.);
#3598=ORIENTED_EDGE('',*,*,#2884,.F.);
#3599=ORIENTED_EDGE('',*,*,#2880,.F.);
#3600=ORIENTED_EDGE('',*,*,#2885,.F.);
#3601=ORIENTED_EDGE('',*,*,#2886,.T.);
#3602=ORIENTED_EDGE('',*,*,#2887,.F.);
#3603=ORIENTED_EDGE('',*,*,#2883,.F.);
#3604=ORIENTED_EDGE('',*,*,#2888,.F.);
#3605=ORIENTED_EDGE('',*,*,#2889,.T.);
#3606=ORIENTED_EDGE('',*,*,#2890,.F.);
#3607=ORIENTED_EDGE('',*,*,#2886,.F.);
#3608=ORIENTED_EDGE('',*,*,#2891,.F.);
#3609=ORIENTED_EDGE('',*,*,#2892,.F.);
#3610=ORIENTED_EDGE('',*,*,#2893,.F.);
#3611=ORIENTED_EDGE('',*,*,#2889,.F.);
#3612=ORIENTED_EDGE('',*,*,#2894,.F.);
#3613=ORIENTED_EDGE('',*,*,#2895,.T.);
#3614=ORIENTED_EDGE('',*,*,#2896,.F.);
#3615=ORIENTED_EDGE('',*,*,#2895,.F.);
#3616=ORIENTED_EDGE('',*,*,#2808,.T.);
#3617=ORIENTED_EDGE('',*,*,#2897,.T.);
#3618=ORIENTED_EDGE('',*,*,#2898,.T.);
#3619=ORIENTED_EDGE('',*,*,#2899,.F.);
#3620=ORIENTED_EDGE('',*,*,#2785,.T.);
#3621=ORIENTED_EDGE('',*,*,#2900,.F.);
#3622=ORIENTED_EDGE('',*,*,#2901,.F.);
#3623=ORIENTED_EDGE('',*,*,#2902,.T.);
#3624=ORIENTED_EDGE('',*,*,#2836,.T.);
#3625=ORIENTED_EDGE('',*,*,#2903,.T.);
#3626=ORIENTED_EDGE('',*,*,#2901,.T.);
#3627=ORIENTED_EDGE('',*,*,#2904,.F.);
#3628=ORIENTED_EDGE('',*,*,#2813,.T.);
#3629=ORIENTED_EDGE('',*,*,#2905,.F.);
#3630=ORIENTED_EDGE('',*,*,#2906,.F.);
#3631=ORIENTED_EDGE('',*,*,#2907,.T.);
#3632=ORIENTED_EDGE('',*,*,#2864,.T.);
#3633=ORIENTED_EDGE('',*,*,#2908,.T.);
#3634=ORIENTED_EDGE('',*,*,#2906,.T.);
#3635=ORIENTED_EDGE('',*,*,#2909,.F.);
#3636=ORIENTED_EDGE('',*,*,#2841,.T.);
#3637=ORIENTED_EDGE('',*,*,#2910,.F.);
#3638=ORIENTED_EDGE('',*,*,#2911,.F.);
#3639=ORIENTED_EDGE('',*,*,#2912,.T.);
#3640=ORIENTED_EDGE('',*,*,#2892,.T.);
#3641=ORIENTED_EDGE('',*,*,#2913,.T.);
#3642=ORIENTED_EDGE('',*,*,#2911,.T.);
#3643=ORIENTED_EDGE('',*,*,#2914,.F.);
#3644=ORIENTED_EDGE('',*,*,#2869,.T.);
#3645=ORIENTED_EDGE('',*,*,#2915,.F.);
#3646=ORIENTED_EDGE('',*,*,#2898,.F.);
#3647=ORIENTED_EDGE('',*,*,#2916,.T.);
#3648=ORIENTED_EDGE('',*,*,#2784,.T.);
#3649=ORIENTED_EDGE('',*,*,#2788,.T.);
#3650=ORIENTED_EDGE('',*,*,#2791,.T.);
#3651=ORIENTED_EDGE('',*,*,#2794,.T.);
#3652=ORIENTED_EDGE('',*,*,#2797,.T.);
#3653=ORIENTED_EDGE('',*,*,#2800,.T.);
#3654=ORIENTED_EDGE('',*,*,#2803,.T.);
#3655=ORIENTED_EDGE('',*,*,#2806,.T.);
#3656=ORIENTED_EDGE('',*,*,#2809,.T.);
#3657=ORIENTED_EDGE('',*,*,#2899,.T.);
#3658=ORIENTED_EDGE('',*,*,#2915,.T.);
#3659=ORIENTED_EDGE('',*,*,#2868,.T.);
#3660=ORIENTED_EDGE('',*,*,#2872,.T.);
#3661=ORIENTED_EDGE('',*,*,#2875,.T.);
#3662=ORIENTED_EDGE('',*,*,#2878,.T.);
#3663=ORIENTED_EDGE('',*,*,#2881,.T.);
#3664=ORIENTED_EDGE('',*,*,#2884,.T.);
#3665=ORIENTED_EDGE('',*,*,#2887,.T.);
#3666=ORIENTED_EDGE('',*,*,#2890,.T.);
#3667=ORIENTED_EDGE('',*,*,#2893,.T.);
#3668=ORIENTED_EDGE('',*,*,#2914,.T.);
#3669=ORIENTED_EDGE('',*,*,#2910,.T.);
#3670=ORIENTED_EDGE('',*,*,#2840,.T.);
#3671=ORIENTED_EDGE('',*,*,#2844,.T.);
#3672=ORIENTED_EDGE('',*,*,#2847,.T.);
#3673=ORIENTED_EDGE('',*,*,#2850,.T.);
#3674=ORIENTED_EDGE('',*,*,#2853,.T.);
#3675=ORIENTED_EDGE('',*,*,#2856,.T.);
#3676=ORIENTED_EDGE('',*,*,#2859,.T.);
#3677=ORIENTED_EDGE('',*,*,#2862,.T.);
#3678=ORIENTED_EDGE('',*,*,#2865,.T.);
#3679=ORIENTED_EDGE('',*,*,#2909,.T.);
#3680=ORIENTED_EDGE('',*,*,#2905,.T.);
#3681=ORIENTED_EDGE('',*,*,#2812,.T.);
#3682=ORIENTED_EDGE('',*,*,#2816,.T.);
#3683=ORIENTED_EDGE('',*,*,#2819,.T.);
#3684=ORIENTED_EDGE('',*,*,#2822,.T.);
#3685=ORIENTED_EDGE('',*,*,#2825,.T.);
#3686=ORIENTED_EDGE('',*,*,#2828,.T.);
#3687=ORIENTED_EDGE('',*,*,#2831,.T.);
#3688=ORIENTED_EDGE('',*,*,#2834,.T.);
#3689=ORIENTED_EDGE('',*,*,#2837,.T.);
#3690=ORIENTED_EDGE('',*,*,#2904,.T.);
#3691=ORIENTED_EDGE('',*,*,#2900,.T.);
#3692=ORIENTED_EDGE('',*,*,#2896,.T.);
#3693=ORIENTED_EDGE('',*,*,#2782,.T.);
#3694=ORIENTED_EDGE('',*,*,#2902,.F.);
#3695=ORIENTED_EDGE('',*,*,#2903,.F.);
#3696=ORIENTED_EDGE('',*,*,#2835,.T.);
#3697=ORIENTED_EDGE('',*,*,#2832,.T.);
#3698=ORIENTED_EDGE('',*,*,#2829,.T.);
#3699=ORIENTED_EDGE('',*,*,#2826,.T.);
#3700=ORIENTED_EDGE('',*,*,#2823,.T.);
#3701=ORIENTED_EDGE('',*,*,#2820,.T.);
#3702=ORIENTED_EDGE('',*,*,#2817,.T.);
#3703=ORIENTED_EDGE('',*,*,#2814,.T.);
#3704=ORIENTED_EDGE('',*,*,#2810,.T.);
#3705=ORIENTED_EDGE('',*,*,#2907,.F.);
#3706=ORIENTED_EDGE('',*,*,#2908,.F.);
#3707=ORIENTED_EDGE('',*,*,#2863,.T.);
#3708=ORIENTED_EDGE('',*,*,#2860,.T.);
#3709=ORIENTED_EDGE('',*,*,#2857,.T.);
#3710=ORIENTED_EDGE('',*,*,#2854,.T.);
#3711=ORIENTED_EDGE('',*,*,#2851,.T.);
#3712=ORIENTED_EDGE('',*,*,#2848,.T.);
#3713=ORIENTED_EDGE('',*,*,#2845,.T.);
#3714=ORIENTED_EDGE('',*,*,#2842,.T.);
#3715=ORIENTED_EDGE('',*,*,#2838,.T.);
#3716=ORIENTED_EDGE('',*,*,#2912,.F.);
#3717=ORIENTED_EDGE('',*,*,#2913,.F.);
#3718=ORIENTED_EDGE('',*,*,#2891,.T.);
#3719=ORIENTED_EDGE('',*,*,#2888,.T.);
#3720=ORIENTED_EDGE('',*,*,#2885,.T.);
#3721=ORIENTED_EDGE('',*,*,#2882,.T.);
#3722=ORIENTED_EDGE('',*,*,#2879,.T.);
#3723=ORIENTED_EDGE('',*,*,#2876,.T.);
#3724=ORIENTED_EDGE('',*,*,#2873,.T.);
#3725=ORIENTED_EDGE('',*,*,#2870,.T.);
#3726=ORIENTED_EDGE('',*,*,#2866,.T.);
#3727=ORIENTED_EDGE('',*,*,#2916,.F.);
#3728=ORIENTED_EDGE('',*,*,#2897,.F.);
#3729=ORIENTED_EDGE('',*,*,#2807,.T.);
#3730=ORIENTED_EDGE('',*,*,#2804,.T.);
#3731=ORIENTED_EDGE('',*,*,#2801,.T.);
#3732=ORIENTED_EDGE('',*,*,#2798,.T.);
#3733=ORIENTED_EDGE('',*,*,#2795,.T.);
#3734=ORIENTED_EDGE('',*,*,#2792,.T.);
#3735=ORIENTED_EDGE('',*,*,#2789,.T.);
#3736=ORIENTED_EDGE('',*,*,#2786,.T.);
#3737=ORIENTED_EDGE('',*,*,#2894,.T.);
#4638=CYLINDRICAL_SURFACE('',#5250,0.21);
#4696=ADVANCED_FACE('',(#597),#386,.F.);
#4697=ADVANCED_FACE('',(#598),#387,.F.);
#4698=ADVANCED_FACE('',(#599),#388,.F.);
#4699=ADVANCED_FACE('',(#600),#389,.F.);
#4700=ADVANCED_FACE('',(#601),#390,.F.);
#4701=ADVANCED_FACE('',(#602),#391,.F.);
#4702=ADVANCED_FACE('',(#603),#392,.F.);
#4703=ADVANCED_FACE('',(#604),#393,.F.);
#4704=ADVANCED_FACE('',(#605),#394,.F.);
#4705=ADVANCED_FACE('',(#606),#395,.F.);
#4706=ADVANCED_FACE('',(#607),#396,.F.);
#4707=ADVANCED_FACE('',(#608),#397,.F.);
#4708=ADVANCED_FACE('',(#609),#398,.F.);
#4709=ADVANCED_FACE('',(#610),#399,.F.);
#4710=ADVANCED_FACE('',(#611),#400,.F.);
#4711=ADVANCED_FACE('',(#612),#401,.F.);
#4712=ADVANCED_FACE('',(#613),#402,.F.);
#4713=ADVANCED_FACE('',(#614),#403,.F.);
#4714=ADVANCED_FACE('',(#615),#404,.F.);
#4715=ADVANCED_FACE('',(#616),#405,.F.);
#4716=ADVANCED_FACE('',(#617),#406,.F.);
#4717=ADVANCED_FACE('',(#618),#407,.F.);
#4718=ADVANCED_FACE('',(#619),#408,.F.);
#4719=ADVANCED_FACE('',(#620),#409,.F.);
#4720=ADVANCED_FACE('',(#621),#410,.F.);
#4721=ADVANCED_FACE('',(#622),#411,.F.);
#4722=ADVANCED_FACE('',(#623),#412,.F.);
#4723=ADVANCED_FACE('',(#624),#413,.F.);
#4724=ADVANCED_FACE('',(#625),#414,.F.);
#4725=ADVANCED_FACE('',(#626),#415,.F.);
#4726=ADVANCED_FACE('',(#627),#416,.F.);
#4727=ADVANCED_FACE('',(#628),#417,.F.);
#4728=ADVANCED_FACE('',(#629),#418,.F.);
#4729=ADVANCED_FACE('',(#630),#419,.F.);
#4730=ADVANCED_FACE('',(#631),#420,.F.);
#4731=ADVANCED_FACE('',(#632),#421,.F.);
#4732=ADVANCED_FACE('',(#633),#4638,.F.);
#4733=ADVANCED_FACE('',(#634),#422,.T.);
#4734=ADVANCED_FACE('',(#635),#423,.T.);
#4735=ADVANCED_FACE('',(#636),#424,.T.);
#4736=ADVANCED_FACE('',(#637),#425,.T.);
#4737=ADVANCED_FACE('',(#638),#426,.T.);
#4738=ADVANCED_FACE('',(#639),#427,.T.);
#4739=ADVANCED_FACE('',(#640),#428,.T.);
#4740=ADVANCED_FACE('',(#641),#429,.T.);
#4741=ADVANCED_FACE('',(#642,#333),#430,.T.);
#4742=ADVANCED_FACE('',(#643,#334),#431,.F.);
#4942=CLOSED_SHELL('',(#4696,#4697,#4698,#4699,#4700,#4701,#4702,#4703,
#4704,#4705,#4706,#4707,#4708,#4709,#4710,#4711,#4712,#4713,#4714,#4715,
#4716,#4717,#4718,#4719,#4720,#4721,#4722,#4723,#4724,#4725,#4726,#4727,
#4728,#4729,#4730,#4731,#4732,#4733,#4734,#4735,#4736,#4737,#4738,#4739,
#4740,#4741,#4742));
#5213=AXIS2_PLACEMENT_3D('',#7182,#5759,#5760);
#5214=AXIS2_PLACEMENT_3D('',#7183,#5761,#5762);
#5215=AXIS2_PLACEMENT_3D('',#7192,#5767,#5768);
#5216=AXIS2_PLACEMENT_3D('',#7198,#5772,#5773);
#5217=AXIS2_PLACEMENT_3D('',#7204,#5777,#5778);
#5218=AXIS2_PLACEMENT_3D('',#7210,#5782,#5783);
#5219=AXIS2_PLACEMENT_3D('',#7216,#5787,#5788);
#5220=AXIS2_PLACEMENT_3D('',#7222,#5792,#5793);
#5221=AXIS2_PLACEMENT_3D('',#7228,#5797,#5798);
#5222=AXIS2_PLACEMENT_3D('',#7234,#5802,#5803);
#5223=AXIS2_PLACEMENT_3D('',#7240,#5807,#5808);
#5224=AXIS2_PLACEMENT_3D('',#7249,#5813,#5814);
#5225=AXIS2_PLACEMENT_3D('',#7255,#5818,#5819);
#5226=AXIS2_PLACEMENT_3D('',#7261,#5823,#5824);
#5227=AXIS2_PLACEMENT_3D('',#7267,#5828,#5829);
#5228=AXIS2_PLACEMENT_3D('',#7273,#5833,#5834);
#5229=AXIS2_PLACEMENT_3D('',#7279,#5838,#5839);
#5230=AXIS2_PLACEMENT_3D('',#7285,#5843,#5844);
#5231=AXIS2_PLACEMENT_3D('',#7291,#5848,#5849);
#5232=AXIS2_PLACEMENT_3D('',#7297,#5853,#5854);
#5233=AXIS2_PLACEMENT_3D('',#7306,#5859,#5860);
#5234=AXIS2_PLACEMENT_3D('',#7312,#5864,#5865);
#5235=AXIS2_PLACEMENT_3D('',#7318,#5869,#5870);
#5236=AXIS2_PLACEMENT_3D('',#7324,#5874,#5875);
#5237=AXIS2_PLACEMENT_3D('',#7330,#5879,#5880);
#5238=AXIS2_PLACEMENT_3D('',#7336,#5884,#5885);
#5239=AXIS2_PLACEMENT_3D('',#7342,#5889,#5890);
#5240=AXIS2_PLACEMENT_3D('',#7348,#5894,#5895);
#5241=AXIS2_PLACEMENT_3D('',#7354,#5899,#5900);
#5242=AXIS2_PLACEMENT_3D('',#7363,#5905,#5906);
#5243=AXIS2_PLACEMENT_3D('',#7369,#5910,#5911);
#5244=AXIS2_PLACEMENT_3D('',#7375,#5915,#5916);
#5245=AXIS2_PLACEMENT_3D('',#7381,#5920,#5921);
#5246=AXIS2_PLACEMENT_3D('',#7387,#5925,#5926);
#5247=AXIS2_PLACEMENT_3D('',#7393,#5930,#5931);
#5248=AXIS2_PLACEMENT_3D('',#7399,#5935,#5936);
#5249=AXIS2_PLACEMENT_3D('',#7405,#5940,#5941);
#5250=AXIS2_PLACEMENT_3D('',#7411,#5945,#5946);
#5251=AXIS2_PLACEMENT_3D('',#7413,#5947,#5948);
#5252=AXIS2_PLACEMENT_3D('',#7416,#5950,#5951);
#5253=AXIS2_PLACEMENT_3D('',#7417,#5952,#5953);
#5254=AXIS2_PLACEMENT_3D('',#7423,#5957,#5958);
#5255=AXIS2_PLACEMENT_3D('',#7429,#5962,#5963);
#5256=AXIS2_PLACEMENT_3D('',#7432,#5966,#5967);
#5257=AXIS2_PLACEMENT_3D('',#7438,#5971,#5972);
#5258=AXIS2_PLACEMENT_3D('',#7441,#5975,#5976);
#5259=AXIS2_PLACEMENT_3D('',#7447,#5980,#5981);
#5260=AXIS2_PLACEMENT_3D('',#7450,#5984,#5985);
#5261=AXIS2_PLACEMENT_3D('',#7453,#5988,#5989);
#5262=AXIS2_PLACEMENT_3D('',#7454,#5990,#5991);
#5759=DIRECTION('axis',(0.,0.,1.));
#5760=DIRECTION('refdir',(1.,0.,0.));
#5761=DIRECTION('center_axis',(0.,0.,-1.));
#5762=DIRECTION('ref_axis',(0.,1.,0.));
#5763=DIRECTION('',(0.,1.,0.));
#5764=DIRECTION('',(1.,0.,0.));
#5765=DIRECTION('',(0.,-1.,0.));
#5766=DIRECTION('',(1.,0.,0.));
#5767=DIRECTION('center_axis',(0.,1.,-8.88178419700125E-16));
#5768=DIRECTION('ref_axis',(0.,8.88178419700125E-16,1.));
#5769=DIRECTION('',(0.,8.88178419700125E-16,1.));
#5770=DIRECTION('',(1.,0.,0.));
#5771=DIRECTION('',(0.,-8.88178419700125E-16,-1.));
#5772=DIRECTION('center_axis',(0.,-7.40148683083439E-16,-1.));
#5773=DIRECTION('ref_axis',(0.,1.,-7.40148683083439E-16));
#5774=DIRECTION('',(0.,1.,-7.40148683083439E-16));
#5775=DIRECTION('',(1.,0.,0.));
#5776=DIRECTION('',(0.,-1.,7.40148683083439E-16));
#5777=DIRECTION('center_axis',(0.,-0.707106781186547,-0.707106781186548));
#5778=DIRECTION('ref_axis',(0.,0.707106781186548,-0.707106781186547));
#5779=DIRECTION('',(0.,0.707106781186548,-0.707106781186547));
#5780=DIRECTION('',(1.,0.,0.));
#5781=DIRECTION('',(0.,-0.707106781186548,0.707106781186547));
#5782=DIRECTION('center_axis',(0.,-1.,2.77555756156289E-16));
#5783=DIRECTION('ref_axis',(0.,-2.77555756156289E-16,-1.));
#5784=DIRECTION('',(0.,-2.77555756156289E-16,-1.));
#5785=DIRECTION('',(1.,0.,0.));
#5786=DIRECTION('',(0.,2.77555756156289E-16,1.));
#5787=DIRECTION('center_axis',(0.,-0.707106781186547,0.707106781186548));
#5788=DIRECTION('ref_axis',(0.,-0.707106781186548,-0.707106781186547));
#5789=DIRECTION('',(0.,-0.707106781186548,-0.707106781186547));
#5790=DIRECTION('',(1.,0.,0.));
#5791=DIRECTION('',(0.,0.707106781186548,0.707106781186547));
#5792=DIRECTION('center_axis',(0.,7.40148683083438E-16,1.));
#5793=DIRECTION('ref_axis',(0.,-1.,7.40148683083438E-16));
#5794=DIRECTION('',(0.,-1.,7.40148683083438E-16));
#5795=DIRECTION('',(1.,0.,0.));
#5796=DIRECTION('',(0.,1.,-7.40148683083438E-16));
#5797=DIRECTION('center_axis',(0.,1.,-4.44089209850063E-16));
#5798=DIRECTION('ref_axis',(0.,4.44089209850063E-16,1.));
#5799=DIRECTION('',(0.,4.44089209850063E-16,1.));
#5800=DIRECTION('',(1.,0.,0.));
#5801=DIRECTION('',(0.,-4.44089209850063E-16,-1.));
#5802=DIRECTION('center_axis',(0.,2.41352831440251E-16,1.));
#5803=DIRECTION('ref_axis',(0.,-1.,2.41352831440251E-16));
#5804=DIRECTION('',(0.,-1.,2.41352831440251E-16));
#5805=DIRECTION('',(-1.,0.,0.));
#5806=DIRECTION('',(0.,1.,-2.41352831440251E-16));
#5807=DIRECTION('center_axis',(0.,-1.,2.41352831440251E-16));
#5808=DIRECTION('ref_axis',(0.,-2.41352831440251E-16,-1.));
#5809=DIRECTION('',(0.,-2.41352831440251E-16,-1.));
#5810=DIRECTION('',(1.,0.,0.));
#5811=DIRECTION('',(0.,2.41352831440251E-16,1.));
#5812=DIRECTION('',(1.,0.,0.));
#5813=DIRECTION('center_axis',(0.,0.,-1.));
#5814=DIRECTION('ref_axis',(0.,1.,0.));
#5815=DIRECTION('',(0.,1.,0.));
#5816=DIRECTION('',(1.,0.,0.));
#5817=DIRECTION('',(0.,-1.,0.));
#5818=DIRECTION('center_axis',(0.,-1.,0.));
#5819=DIRECTION('ref_axis',(0.,0.,-1.));
#5820=DIRECTION('',(0.,0.,-1.));
#5821=DIRECTION('',(1.,0.,0.));
#5822=DIRECTION('',(0.,0.,1.));
#5823=DIRECTION('center_axis',(0.,-0.707106781186547,0.707106781186548));
#5824=DIRECTION('ref_axis',(0.,-0.707106781186548,-0.707106781186547));
#5825=DIRECTION('',(0.,-0.707106781186548,-0.707106781186547));
#5826=DIRECTION('',(1.,0.,0.));
#5827=DIRECTION('',(0.,0.707106781186548,0.707106781186547));
#5828=DIRECTION('center_axis',(0.,0.,1.));
#5829=DIRECTION('ref_axis',(0.,-1.,0.));
#5830=DIRECTION('',(0.,-1.,0.));
#5831=DIRECTION('',(1.,0.,0.));
#5832=DIRECTION('',(0.,1.,0.));
#5833=DIRECTION('center_axis',(0.,0.707106781186548,0.707106781186547));
#5834=DIRECTION('ref_axis',(0.,-0.707106781186547,0.707106781186548));
#5835=DIRECTION('',(0.,-0.707106781186547,0.707106781186548));
#5836=DIRECTION('',(1.,0.,0.));
#5837=DIRECTION('',(0.,0.707106781186547,-0.707106781186548));
#5838=DIRECTION('center_axis',(0.,1.,0.));
#5839=DIRECTION('ref_axis',(0.,0.,1.));
#5840=DIRECTION('',(0.,0.,1.));
#5841=DIRECTION('',(1.,0.,0.));
#5842=DIRECTION('',(0.,0.,-1.));
#5843=DIRECTION('center_axis',(0.,0.,-1.));
#5844=DIRECTION('ref_axis',(0.,1.,0.));
#5845=DIRECTION('',(0.,1.,0.));
#5846=DIRECTION('',(1.,0.,0.));
#5847=DIRECTION('',(0.,-1.,0.));
#5848=DIRECTION('center_axis',(0.,1.,-2.41352831440251E-16));
#5849=DIRECTION('ref_axis',(0.,2.41352831440251E-16,1.));
#5850=DIRECTION('',(0.,2.41352831440251E-16,1.));
#5851=DIRECTION('',(-1.,0.,0.));
#5852=DIRECTION('',(0.,-2.41352831440251E-16,-1.));
#5853=DIRECTION('center_axis',(0.,0.,1.));
#5854=DIRECTION('ref_axis',(0.,-1.,0.));
#5855=DIRECTION('',(0.,-1.,0.));
#5856=DIRECTION('',(1.,0.,0.));
#5857=DIRECTION('',(0.,1.,0.));
#5858=DIRECTION('',(1.,0.,0.));
#5859=DIRECTION('center_axis',(0.,-1.,0.));
#5860=DIRECTION('ref_axis',(0.,0.,-1.));
#5861=DIRECTION('',(0.,0.,-1.));
#5862=DIRECTION('',(1.,0.,0.));
#5863=DIRECTION('',(0.,0.,1.));
#5864=DIRECTION('center_axis',(0.,0.,1.));
#5865=DIRECTION('ref_axis',(0.,-1.,0.));
#5866=DIRECTION('',(0.,-1.,0.));
#5867=DIRECTION('',(1.,0.,0.));
#5868=DIRECTION('',(0.,1.,0.));
#5869=DIRECTION('center_axis',(0.,0.707106781186548,0.707106781186548));
#5870=DIRECTION('ref_axis',(0.,-0.707106781186548,0.707106781186548));
#5871=DIRECTION('',(0.,-0.707106781186548,0.707106781186548));
#5872=DIRECTION('',(1.,0.,0.));
#5873=DIRECTION('',(0.,0.707106781186548,-0.707106781186548));
#5874=DIRECTION('center_axis',(0.,1.,0.));
#5875=DIRECTION('ref_axis',(0.,0.,1.));
#5876=DIRECTION('',(0.,0.,1.));
#5877=DIRECTION('',(1.,0.,0.));
#5878=DIRECTION('',(0.,0.,-1.));
#5879=DIRECTION('center_axis',(0.,0.707106781186548,-0.707106781186547));
#5880=DIRECTION('ref_axis',(0.,0.707106781186547,0.707106781186548));
#5881=DIRECTION('',(0.,0.707106781186547,0.707106781186548));
#5882=DIRECTION('',(1.,0.,0.));
#5883=DIRECTION('',(0.,-0.707106781186547,-0.707106781186548));
#5884=DIRECTION('center_axis',(0.,-7.40148683083438E-16,-1.));
#5885=DIRECTION('ref_axis',(0.,1.,-7.40148683083438E-16));
#5886=DIRECTION('',(0.,1.,-7.40148683083438E-16));
#5887=DIRECTION('',(1.,0.,0.));
#5888=DIRECTION('',(0.,-1.,7.40148683083438E-16));
#5889=DIRECTION('center_axis',(0.,-1.,0.));
#5890=DIRECTION('ref_axis',(0.,0.,-1.));
#5891=DIRECTION('',(0.,0.,-1.));
#5892=DIRECTION('',(1.,0.,0.));
#5893=DIRECTION('',(0.,0.,1.));
#5894=DIRECTION('center_axis',(0.,0.,-1.));
#5895=DIRECTION('ref_axis',(0.,1.,0.));
#5896=DIRECTION('',(0.,1.,0.));
#5897=DIRECTION('',(-1.,0.,0.));
#5898=DIRECTION('',(0.,-1.,0.));
#5899=DIRECTION('center_axis',(0.,1.,0.));
#5900=DIRECTION('ref_axis',(0.,0.,1.));
#5901=DIRECTION('',(0.,0.,1.));
#5902=DIRECTION('',(1.,0.,0.));
#5903=DIRECTION('',(0.,0.,-1.));
#5904=DIRECTION('',(1.,0.,0.));
#5905=DIRECTION('center_axis',(0.,0.,1.));
#5906=DIRECTION('ref_axis',(0.,-1.,0.));
#5907=DIRECTION('',(0.,-1.,0.));
#5908=DIRECTION('',(1.,0.,0.));
#5909=DIRECTION('',(0.,1.,0.));
#5910=DIRECTION('center_axis',(0.,1.,0.));
#5911=DIRECTION('ref_axis',(0.,0.,1.));
#5912=DIRECTION('',(0.,0.,1.));
#5913=DIRECTION('',(1.,0.,0.));
#5914=DIRECTION('',(0.,0.,-1.));
#5915=DIRECTION('center_axis',(0.,0.707106781186547,-0.707106781186548));
#5916=DIRECTION('ref_axis',(0.,0.707106781186548,0.707106781186547));
#5917=DIRECTION('',(0.,0.707106781186548,0.707106781186547));
#5918=DIRECTION('',(1.,0.,0.));
#5919=DIRECTION('',(0.,-0.707106781186548,-0.707106781186547));
#5920=DIRECTION('center_axis',(0.,0.,-1.));
#5921=DIRECTION('ref_axis',(0.,1.,0.));
#5922=DIRECTION('',(0.,1.,0.));
#5923=DIRECTION('',(1.,0.,0.));
#5924=DIRECTION('',(0.,-1.,0.));
#5925=DIRECTION('center_axis',(0.,-0.707106781186547,-0.707106781186548));
#5926=DIRECTION('ref_axis',(0.,0.707106781186548,-0.707106781186547));
#5927=DIRECTION('',(0.,0.707106781186548,-0.707106781186547));
#5928=DIRECTION('',(1.,0.,0.));
#5929=DIRECTION('',(0.,-0.707106781186548,0.707106781186547));
#5930=DIRECTION('center_axis',(0.,-1.,0.));
#5931=DIRECTION('ref_axis',(0.,0.,-1.));
#5932=DIRECTION('',(0.,0.,-1.));
#5933=DIRECTION('',(1.,0.,0.));
#5934=DIRECTION('',(0.,0.,1.));
#5935=DIRECTION('center_axis',(0.,0.,1.));
#5936=DIRECTION('ref_axis',(0.,-1.,0.));
#5937=DIRECTION('',(0.,-1.,0.));
#5938=DIRECTION('',(1.,0.,0.));
#5939=DIRECTION('',(0.,1.,0.));
#5940=DIRECTION('center_axis',(0.,-1.,0.));
#5941=DIRECTION('ref_axis',(0.,0.,-1.));
#5942=DIRECTION('',(0.,0.,-1.));
#5943=DIRECTION('',(-1.,0.,0.));
#5944=DIRECTION('',(0.,0.,1.));
#5945=DIRECTION('center_axis',(1.,0.,0.));
#5946=DIRECTION('ref_axis',(0.,0.,-1.));
#5947=DIRECTION('center_axis',(1.,0.,0.));
#5948=DIRECTION('ref_axis',(0.,0.,-1.));
#5949=DIRECTION('',(1.,0.,0.));
#5950=DIRECTION('center_axis',(-1.,0.,0.));
#5951=DIRECTION('ref_axis',(0.,0.,-1.));
#5952=DIRECTION('center_axis',(0.,1.,0.));
#5953=DIRECTION('ref_axis',(0.,0.,1.));
#5954=DIRECTION('',(0.,0.,1.));
#5955=DIRECTION('',(1.,0.,0.));
#5956=DIRECTION('',(0.,0.,1.));
#5957=DIRECTION('center_axis',(0.,1.,0.));
#5958=DIRECTION('ref_axis',(0.,0.,1.));
#5959=DIRECTION('',(0.,0.,1.));
#5960=DIRECTION('',(1.,0.,0.));
#5961=DIRECTION('',(0.,0.,1.));
#5962=DIRECTION('center_axis',(0.,0.,-1.));
#5963=DIRECTION('ref_axis',(0.,1.,0.));
#5964=DIRECTION('',(0.,1.,0.));
#5965=DIRECTION('',(0.,1.,0.));
#5966=DIRECTION('center_axis',(0.,0.,-1.));
#5967=DIRECTION('ref_axis',(0.,1.,0.));
#5968=DIRECTION('',(0.,1.,0.));
#5969=DIRECTION('',(1.,0.,0.));
#5970=DIRECTION('',(0.,1.,0.));
#5971=DIRECTION('center_axis',(0.,-1.,0.));
#5972=DIRECTION('ref_axis',(0.,0.,-1.));
#5973=DIRECTION('',(0.,0.,-1.));
#5974=DIRECTION('',(0.,0.,-1.));
#5975=DIRECTION('center_axis',(0.,-1.,0.));
#5976=DIRECTION('ref_axis',(0.,0.,-1.));
#5977=DIRECTION('',(0.,0.,-1.));
#5978=DIRECTION('',(1.,0.,0.));
#5979=DIRECTION('',(0.,0.,-1.));
#5980=DIRECTION('center_axis',(0.,0.,1.));
#5981=DIRECTION('ref_axis',(0.,-1.,0.));
#5982=DIRECTION('',(0.,-1.,0.));
#5983=DIRECTION('',(0.,-1.,0.));
#5984=DIRECTION('center_axis',(0.,0.,1.));
#5985=DIRECTION('ref_axis',(0.,-1.,0.));
#5986=DIRECTION('',(0.,-1.,0.));
#5987=DIRECTION('',(0.,-1.,0.));
#5988=DIRECTION('center_axis',(1.,0.,0.));
#5989=DIRECTION('ref_axis',(0.,0.,-1.));
#5990=DIRECTION('center_axis',(1.,0.,0.));
#5991=DIRECTION('ref_axis',(0.,0.,-1.));
#7182=CARTESIAN_POINT('',(0.,0.,0.));
#7183=CARTESIAN_POINT('Origin',(-0.1,0.82,-0.3));
#7184=CARTESIAN_POINT('',(0.,0.82,-0.3));
#7185=CARTESIAN_POINT('',(0.,1.,-0.3));
#7186=CARTESIAN_POINT('',(0.,0.41,-0.3));
#7187=CARTESIAN_POINT('',(30.,0.82,-0.3));
#7188=CARTESIAN_POINT('',(-0.1,0.82,-0.3));
#7189=CARTESIAN_POINT('',(30.,1.,-0.3));
#7190=CARTESIAN_POINT('',(30.,0.41,-0.3));
#7191=CARTESIAN_POINT('',(-0.05,1.,-0.3));
#7192=CARTESIAN_POINT('Origin',(-0.1,0.82,-0.55));
#7193=CARTESIAN_POINT('',(0.,0.82,-0.55));
#7194=CARTESIAN_POINT('',(0.,0.82,-0.275));
#7195=CARTESIAN_POINT('',(30.,0.82,-0.55));
#7196=CARTESIAN_POINT('',(-0.1,0.82,-0.55));
#7197=CARTESIAN_POINT('',(30.,0.82,-0.275));
#7198=CARTESIAN_POINT('Origin',(-0.1,0.67,-0.55));
#7199=CARTESIAN_POINT('',(0.,0.67,-0.55));
#7200=CARTESIAN_POINT('',(0.,0.335,-0.55));
#7201=CARTESIAN_POINT('',(30.,0.67,-0.55));
#7202=CARTESIAN_POINT('',(-0.1,0.67,-0.55));
#7203=CARTESIAN_POINT('',(30.,0.335,-0.55));
#7204=CARTESIAN_POINT('Origin',(-0.1,0.42,-0.3));
#7205=CARTESIAN_POINT('',(0.,0.42,-0.3));
#7206=CARTESIAN_POINT('',(0.,0.24,-0.12));
#7207=CARTESIAN_POINT('',(30.,0.42,-0.3));
#7208=CARTESIAN_POINT('',(-0.1,0.42,-0.3));
#7209=CARTESIAN_POINT('',(30.,0.24,-0.12));
#7210=CARTESIAN_POINT('Origin',(-0.1,0.42,0.3));
#7211=CARTESIAN_POINT('',(0.,0.42,0.3));
#7212=CARTESIAN_POINT('',(0.,0.42,0.15));
#7213=CARTESIAN_POINT('',(30.,0.42,0.3));
#7214=CARTESIAN_POINT('',(-0.1,0.42,0.3));
#7215=CARTESIAN_POINT('',(30.,0.42,0.15));
#7216=CARTESIAN_POINT('Origin',(-0.1,0.67,0.55));
#7217=CARTESIAN_POINT('',(0.,0.67,0.55));
#7218=CARTESIAN_POINT('',(6.93889390390723E-18,0.365,0.245));
#7219=CARTESIAN_POINT('',(30.,0.67,0.55));
#7220=CARTESIAN_POINT('',(-0.1,0.67,0.55));
#7221=CARTESIAN_POINT('',(30.,0.365,0.245));
#7222=CARTESIAN_POINT('Origin',(-0.1,0.82,0.55));
#7223=CARTESIAN_POINT('',(0.,0.82,0.55));
#7224=CARTESIAN_POINT('',(0.,0.41,0.55));
#7225=CARTESIAN_POINT('',(30.,0.82,0.55));
#7226=CARTESIAN_POINT('',(-0.1,0.82,0.55));
#7227=CARTESIAN_POINT('',(30.,0.41,0.55));
#7228=CARTESIAN_POINT('Origin',(-0.1,0.82,0.3));
#7229=CARTESIAN_POINT('',(0.,0.82,0.3));
#7230=CARTESIAN_POINT('',(0.,0.82,0.15));
#7231=CARTESIAN_POINT('',(30.,0.82,0.3));
#7232=CARTESIAN_POINT('',(-0.1,0.82,0.3));
#7233=CARTESIAN_POINT('',(30.,0.82,0.15));
#7234=CARTESIAN_POINT('Origin',(-0.1,1.05,0.3));
#7235=CARTESIAN_POINT('',(0.,1.,0.3));
#7236=CARTESIAN_POINT('',(0.,0.525,0.3));
#7237=CARTESIAN_POINT('',(30.,1.,0.3));
#7238=CARTESIAN_POINT('',(-0.05,1.,0.3));
#7239=CARTESIAN_POINT('',(30.,0.525,0.3));
#7240=CARTESIAN_POINT('Origin',(-0.1,-0.3,-0.82));
#7241=CARTESIAN_POINT('',(0.,-0.3,-0.82));
#7242=CARTESIAN_POINT('',(0.,-0.3,-1.));
#7243=CARTESIAN_POINT('',(0.,-0.3,-0.41));
#7244=CARTESIAN_POINT('',(30.,-0.3,-0.82));
#7245=CARTESIAN_POINT('',(-0.1,-0.3,-0.82));
#7246=CARTESIAN_POINT('',(30.,-0.3,-1.));
#7247=CARTESIAN_POINT('',(30.,-0.3,-0.41));
#7248=CARTESIAN_POINT('',(-0.05,-0.3,-1.));
#7249=CARTESIAN_POINT('Origin',(-0.1,-0.55,-0.82));
#7250=CARTESIAN_POINT('',(0.,-0.55,-0.82));
#7251=CARTESIAN_POINT('',(0.,-0.275,-0.82));
#7252=CARTESIAN_POINT('',(30.,-0.55,-0.82));
#7253=CARTESIAN_POINT('',(-0.1,-0.55,-0.82));
#7254=CARTESIAN_POINT('',(30.,-0.275,-0.82));
#7255=CARTESIAN_POINT('Origin',(-0.1,-0.55,-0.67));
#7256=CARTESIAN_POINT('',(0.,-0.55,-0.67));
#7257=CARTESIAN_POINT('',(0.,-0.55,-0.335));
#7258=CARTESIAN_POINT('',(30.,-0.55,-0.67));
#7259=CARTESIAN_POINT('',(-0.1,-0.55,-0.67));
#7260=CARTESIAN_POINT('',(30.,-0.55,-0.335));
#7261=CARTESIAN_POINT('Origin',(-0.1,-0.3,-0.42));
#7262=CARTESIAN_POINT('',(0.,-0.3,-0.42));
#7263=CARTESIAN_POINT('',(0.,-0.12,-0.24));
#7264=CARTESIAN_POINT('',(30.,-0.3,-0.42));
#7265=CARTESIAN_POINT('',(-0.1,-0.3,-0.42));
#7266=CARTESIAN_POINT('',(30.,-0.12,-0.24));
#7267=CARTESIAN_POINT('Origin',(-0.1,0.3,-0.42));
#7268=CARTESIAN_POINT('',(0.,0.3,-0.42));
#7269=CARTESIAN_POINT('',(0.,0.15,-0.42));
#7270=CARTESIAN_POINT('',(30.,0.3,-0.42));
#7271=CARTESIAN_POINT('',(-0.1,0.3,-0.42));
#7272=CARTESIAN_POINT('',(30.,0.15,-0.42));
#7273=CARTESIAN_POINT('Origin',(-0.1,0.55,-0.67));
#7274=CARTESIAN_POINT('',(0.,0.55,-0.67));
#7275=CARTESIAN_POINT('',(0.,0.245,-0.365));
#7276=CARTESIAN_POINT('',(30.,0.55,-0.67));
#7277=CARTESIAN_POINT('',(-0.1,0.55,-0.67));
#7278=CARTESIAN_POINT('',(30.,0.245,-0.365));
#7279=CARTESIAN_POINT('Origin',(-0.1,0.55,-0.82));
#7280=CARTESIAN_POINT('',(0.,0.55,-0.82));
#7281=CARTESIAN_POINT('',(0.,0.55,-0.41));
#7282=CARTESIAN_POINT('',(30.,0.55,-0.82));
#7283=CARTESIAN_POINT('',(-0.1,0.55,-0.82));
#7284=CARTESIAN_POINT('',(30.,0.55,-0.41));
#7285=CARTESIAN_POINT('Origin',(-0.1,0.3,-0.82));
#7286=CARTESIAN_POINT('',(0.,0.3,-0.82));
#7287=CARTESIAN_POINT('',(0.,0.15,-0.82));
#7288=CARTESIAN_POINT('',(30.,0.3,-0.82));
#7289=CARTESIAN_POINT('',(-0.1,0.3,-0.82));
#7290=CARTESIAN_POINT('',(30.,0.15,-0.82));
#7291=CARTESIAN_POINT('Origin',(-0.1,0.3,-1.05));
#7292=CARTESIAN_POINT('',(0.,0.3,-1.));
#7293=CARTESIAN_POINT('',(0.,0.3,-0.525));
#7294=CARTESIAN_POINT('',(30.,0.3,-1.));
#7295=CARTESIAN_POINT('',(-0.05,0.3,-1.));
#7296=CARTESIAN_POINT('',(30.,0.3,-0.525));
#7297=CARTESIAN_POINT('Origin',(-0.1,-0.82,0.3));
#7298=CARTESIAN_POINT('',(0.,-0.82,0.3));
#7299=CARTESIAN_POINT('',(0.,-1.,0.3));
#7300=CARTESIAN_POINT('',(0.,-0.41,0.3));
#7301=CARTESIAN_POINT('',(30.,-0.82,0.3));
#7302=CARTESIAN_POINT('',(-0.1,-0.82,0.3));
#7303=CARTESIAN_POINT('',(30.,-1.,0.3));
#7304=CARTESIAN_POINT('',(30.,-0.41,0.3));
#7305=CARTESIAN_POINT('',(-0.05,-1.,0.3));
#7306=CARTESIAN_POINT('Origin',(-0.1,-0.82,0.55));
#7307=CARTESIAN_POINT('',(0.,-0.82,0.55));
#7308=CARTESIAN_POINT('',(0.,-0.82,0.275));
#7309=CARTESIAN_POINT('',(30.,-0.82,0.55));
#7310=CARTESIAN_POINT('',(-0.1,-0.82,0.55));
#7311=CARTESIAN_POINT('',(30.,-0.82,0.275));
#7312=CARTESIAN_POINT('Origin',(-0.1,-0.67,0.55));
#7313=CARTESIAN_POINT('',(0.,-0.67,0.55));
#7314=CARTESIAN_POINT('',(0.,-0.335,0.55));
#7315=CARTESIAN_POINT('',(30.,-0.67,0.55));
#7316=CARTESIAN_POINT('',(-0.1,-0.67,0.55));
#7317=CARTESIAN_POINT('',(30.,-0.335,0.55));
#7318=CARTESIAN_POINT('Origin',(-0.1,-0.42,0.3));
#7319=CARTESIAN_POINT('',(0.,-0.42,0.3));
#7320=CARTESIAN_POINT('',(-6.93889390390723E-18,-0.24,0.12));
#7321=CARTESIAN_POINT('',(30.,-0.42,0.3));
#7322=CARTESIAN_POINT('',(-0.1,-0.42,0.3));
#7323=CARTESIAN_POINT('',(30.,-0.24,0.12));
#7324=CARTESIAN_POINT('Origin',(-0.1,-0.42,-0.3));
#7325=CARTESIAN_POINT('',(0.,-0.42,-0.3));
#7326=CARTESIAN_POINT('',(0.,-0.42,-0.15));
#7327=CARTESIAN_POINT('',(30.,-0.42,-0.3));
#7328=CARTESIAN_POINT('',(-0.1,-0.42,-0.3));
#7329=CARTESIAN_POINT('',(30.,-0.42,-0.15));
#7330=CARTESIAN_POINT('Origin',(-0.1,-0.67,-0.55));
#7331=CARTESIAN_POINT('',(0.,-0.67,-0.55));
#7332=CARTESIAN_POINT('',(0.,-0.365,-0.245));
#7333=CARTESIAN_POINT('',(30.,-0.67,-0.55));
#7334=CARTESIAN_POINT('',(-0.1,-0.67,-0.55));
#7335=CARTESIAN_POINT('',(30.,-0.365,-0.245));
#7336=CARTESIAN_POINT('Origin',(-0.1,-0.82,-0.55));
#7337=CARTESIAN_POINT('',(0.,-0.82,-0.55));
#7338=CARTESIAN_POINT('',(0.,-0.41,-0.55));
#7339=CARTESIAN_POINT('',(30.,-0.82,-0.55));
#7340=CARTESIAN_POINT('',(-0.1,-0.82,-0.55));
#7341=CARTESIAN_POINT('',(30.,-0.41,-0.55));
#7342=CARTESIAN_POINT('Origin',(-0.1,-0.82,-0.3));
#7343=CARTESIAN_POINT('',(0.,-0.82,-0.3));
#7344=CARTESIAN_POINT('',(0.,-0.82,-0.15));
#7345=CARTESIAN_POINT('',(30.,-0.82,-0.3));
#7346=CARTESIAN_POINT('',(-0.1,-0.82,-0.3));
#7347=CARTESIAN_POINT('',(30.,-0.82,-0.15));
#7348=CARTESIAN_POINT('Origin',(-0.1,-1.05,-0.3));
#7349=CARTESIAN_POINT('',(0.,-1.,-0.3));
#7350=CARTESIAN_POINT('',(0.,-0.525,-0.3));
#7351=CARTESIAN_POINT('',(30.,-1.,-0.3));
#7352=CARTESIAN_POINT('',(-0.05,-1.,-0.3));
#7353=CARTESIAN_POINT('',(30.,-0.525,-0.3));
#7354=CARTESIAN_POINT('Origin',(-0.1,0.3,0.82));
#7355=CARTESIAN_POINT('',(0.,0.3,0.82));
#7356=CARTESIAN_POINT('',(0.,0.3,1.));
#7357=CARTESIAN_POINT('',(0.,0.3,0.41));
#7358=CARTESIAN_POINT('',(30.,0.3,0.82));
#7359=CARTESIAN_POINT('',(-0.1,0.3,0.82));
#7360=CARTESIAN_POINT('',(30.,0.3,1.));
#7361=CARTESIAN_POINT('',(30.,0.3,0.41));
#7362=CARTESIAN_POINT('',(-0.05,0.3,1.));
#7363=CARTESIAN_POINT('Origin',(-0.1,0.55,0.82));
#7364=CARTESIAN_POINT('',(0.,0.55,0.82));
#7365=CARTESIAN_POINT('',(0.,0.275,0.82));
#7366=CARTESIAN_POINT('',(30.,0.55,0.82));
#7367=CARTESIAN_POINT('',(-0.1,0.55,0.82));
#7368=CARTESIAN_POINT('',(30.,0.275,0.82));
#7369=CARTESIAN_POINT('Origin',(-0.1,0.55,0.67));
#7370=CARTESIAN_POINT('',(0.,0.55,0.67));
#7371=CARTESIAN_POINT('',(0.,0.55,0.335));
#7372=CARTESIAN_POINT('',(30.,0.55,0.67));
#7373=CARTESIAN_POINT('',(-0.1,0.55,0.67));
#7374=CARTESIAN_POINT('',(30.,0.55,0.335));
#7375=CARTESIAN_POINT('Origin',(-0.1,0.3,0.42));
#7376=CARTESIAN_POINT('',(0.,0.3,0.42));
#7377=CARTESIAN_POINT('',(6.93889390390723E-18,0.12,0.24));
#7378=CARTESIAN_POINT('',(30.,0.3,0.42));
#7379=CARTESIAN_POINT('',(-0.1,0.3,0.42));
#7380=CARTESIAN_POINT('',(30.,0.12,0.24));
#7381=CARTESIAN_POINT('Origin',(-0.1,-0.3,0.42));
#7382=CARTESIAN_POINT('',(0.,-0.3,0.42));
#7383=CARTESIAN_POINT('',(0.,-0.15,0.42));
#7384=CARTESIAN_POINT('',(30.,-0.3,0.42));
#7385=CARTESIAN_POINT('',(-0.1,-0.3,0.42));
#7386=CARTESIAN_POINT('',(30.,-0.15,0.42));
#7387=CARTESIAN_POINT('Origin',(-0.1,-0.55,0.67));
#7388=CARTESIAN_POINT('',(0.,-0.55,0.67));
#7389=CARTESIAN_POINT('',(6.93889390390723E-18,-0.245,0.365));
#7390=CARTESIAN_POINT('',(30.,-0.55,0.67));
#7391=CARTESIAN_POINT('',(-0.1,-0.55,0.67));
#7392=CARTESIAN_POINT('',(30.,-0.245,0.365));
#7393=CARTESIAN_POINT('Origin',(-0.1,-0.55,0.82));
#7394=CARTESIAN_POINT('',(0.,-0.55,0.82));
#7395=CARTESIAN_POINT('',(0.,-0.55,0.41));
#7396=CARTESIAN_POINT('',(30.,-0.55,0.82));
#7397=CARTESIAN_POINT('',(-0.1,-0.55,0.82));
#7398=CARTESIAN_POINT('',(30.,-0.55,0.41));
#7399=CARTESIAN_POINT('Origin',(-0.1,-0.3,0.82));
#7400=CARTESIAN_POINT('',(0.,-0.3,0.82));
#7401=CARTESIAN_POINT('',(0.,-0.15,0.82));
#7402=CARTESIAN_POINT('',(30.,-0.3,0.82));
#7403=CARTESIAN_POINT('',(-0.1,-0.3,0.82));
#7404=CARTESIAN_POINT('',(30.,-0.15,0.82));
#7405=CARTESIAN_POINT('Origin',(-0.1,-0.3,1.05));
#7406=CARTESIAN_POINT('',(0.,-0.3,1.));
#7407=CARTESIAN_POINT('',(0.,-0.3,0.525));
#7408=CARTESIAN_POINT('',(30.,-0.3,1.));
#7409=CARTESIAN_POINT('',(-0.05,-0.3,1.));
#7410=CARTESIAN_POINT('',(30.,-0.3,0.525));
#7411=CARTESIAN_POINT('Origin',(-0.1,0.,0.));
#7412=CARTESIAN_POINT('',(0.,-2.57175827820944E-17,0.21));
#7413=CARTESIAN_POINT('Origin',(0.,0.,0.));
#7414=CARTESIAN_POINT('',(30.,2.57175827820944E-17,0.21));
#7415=CARTESIAN_POINT('',(-0.1,-2.57175827820944E-17,0.21));
#7416=CARTESIAN_POINT('Origin',(30.,0.,0.));
#7417=CARTESIAN_POINT('Origin',(0.,1.,-1.));
#7418=CARTESIAN_POINT('',(0.,1.,1.));
#7419=CARTESIAN_POINT('',(0.,1.,-1.));
#7420=CARTESIAN_POINT('',(30.,1.,1.));
#7421=CARTESIAN_POINT('',(0.,1.,1.));
#7422=CARTESIAN_POINT('',(30.,1.,-1.));
#7423=CARTESIAN_POINT('Origin',(0.,1.,-1.));
#7424=CARTESIAN_POINT('',(30.,1.,-1.));
#7425=CARTESIAN_POINT('',(30.,1.,-1.));
#7426=CARTESIAN_POINT('',(0.,1.,-1.));
#7427=CARTESIAN_POINT('',(0.,1.,-1.));
#7428=CARTESIAN_POINT('',(0.,1.,-1.));
#7429=CARTESIAN_POINT('Origin',(0.,-1.,-1.));
#7430=CARTESIAN_POINT('',(0.,-1.,-1.));
#7431=CARTESIAN_POINT('',(30.,-1.,-1.));
#7432=CARTESIAN_POINT('Origin',(0.,-1.,-1.));
#7433=CARTESIAN_POINT('',(30.,-1.,-1.));
#7434=CARTESIAN_POINT('',(30.,-1.,-1.));
#7435=CARTESIAN_POINT('',(0.,-1.,-1.));
#7436=CARTESIAN_POINT('',(0.,-1.,-1.));
#7437=CARTESIAN_POINT('',(0.,-1.,-1.));
#7438=CARTESIAN_POINT('Origin',(0.,-1.,1.));
#7439=CARTESIAN_POINT('',(0.,-1.,1.));
#7440=CARTESIAN_POINT('',(30.,-1.,1.));
#7441=CARTESIAN_POINT('Origin',(0.,-1.,1.));
#7442=CARTESIAN_POINT('',(30.,-1.,1.));
#7443=CARTESIAN_POINT('',(30.,-1.,1.));
#7444=CARTESIAN_POINT('',(0.,-1.,1.));
#7445=CARTESIAN_POINT('',(0.,-1.,1.));
#7446=CARTESIAN_POINT('',(0.,-1.,1.));
#7447=CARTESIAN_POINT('Origin',(0.,1.,1.));
#7448=CARTESIAN_POINT('',(0.,1.,1.));
#7449=CARTESIAN_POINT('',(30.,1.,1.));
#7450=CARTESIAN_POINT('Origin',(0.,1.,1.));
#7451=CARTESIAN_POINT('',(30.,1.,1.));
#7452=CARTESIAN_POINT('',(0.,1.,1.));
#7453=CARTESIAN_POINT('Origin',(30.,0.,0.));
#7454=CARTESIAN_POINT('Origin',(0.,0.,0.));
#8457=UNCERTAINTY_MEASURE_WITH_UNIT(LENGTH_MEASURE(0.001),#8500,
'DISTANCE_ACCURACY_VALUE',
'Maximum model space distance between geometric entities at asserted c
onnectivities');
#8476=UNCERTAINTY_MEASURE_WITH_UNIT(LENGTH_MEASURE(0.001),#8500,
'DISTANCE_ACCURACY_VALUE',
'Maximum model space distance between geometric entities at asserted c
onnectivities');
#8480=(
GEOMETRIC_REPRESENTATION_CONTEXT(3)
GLOBAL_UNCERTAINTY_ASSIGNED_CONTEXT((#8457))
GLOBAL_UNIT_ASSIGNED_CONTEXT((#8500,#8502,#8503))
REPRESENTATION_CONTEXT('','3D')
);
#8499=(
GEOMETRIC_REPRESENTATION_CONTEXT(3)
GLOBAL_UNCERTAINTY_ASSIGNED_CONTEXT((#8476))
GLOBAL_UNIT_ASSIGNED_CONTEXT((#8500,#8502,#8503))
REPRESENTATION_CONTEXT('','3D')
);
#8500=(
LENGTH_UNIT()
NAMED_UNIT(*)
SI_UNIT(.CENTI.,.METRE.)
);
#8502=(
NAMED_UNIT(*)
PLANE_ANGLE_UNIT()
SI_UNIT($,.RADIAN.)
);
#8503=(
NAMED_UNIT(*)
SI_UNIT($,.STERADIAN.)
SOLID_ANGLE_UNIT()
);
#8507=SHAPE_DEFINITION_REPRESENTATION(#8529,#8601);
#8529=PRODUCT_DEFINITION_SHAPE('',$,#8624);
#8601=SHAPE_REPRESENTATION('',(#5213),#8480);
#8620=PRODUCT_DEFINITION_CONTEXT('part definition',#8688,'design');
#8624=PRODUCT_DEFINITION('Slotted Extrusion - 20 x 20 x 300 mm',
'Slotted Extrusion - 20 x 20 x 300 mm',#8646,#8620);
#8646=PRODUCT_DEFINITION_FORMATION('',$,#8693);
#8688=APPLICATION_CONTEXT(
'Core Data for Automotive Mechanical Design Process');
#8689=PRODUCT_CONTEXT('part definition',#8688,'mechanical');
#8693=PRODUCT('Slotted Extrusion - 20 x 20 x 300 mm',
'Slotted Extrusion - 20 x 20 x 300 mm',
'Slotted Extrusion - 20 x 20 x 300 mm',(#8689));
#8796=COLOUR_RGB('Off White',0.89,0.88,0.83);
#8797=FILL_AREA_STYLE_COLOUR('',#8796);
#8798=FILL_AREA_STYLE('',(#8797));
#8799=SURFACE_STYLE_FILL_AREA(#8798);
#8800=SURFACE_SIDE_STYLE('',(#8799));
#8801=SURFACE_STYLE_USAGE(.BOTH.,#8800);
#8802=PRESENTATION_STYLE_ASSIGNMENT((#8801));
ENDSEC;
END-ISO-10303-21;
